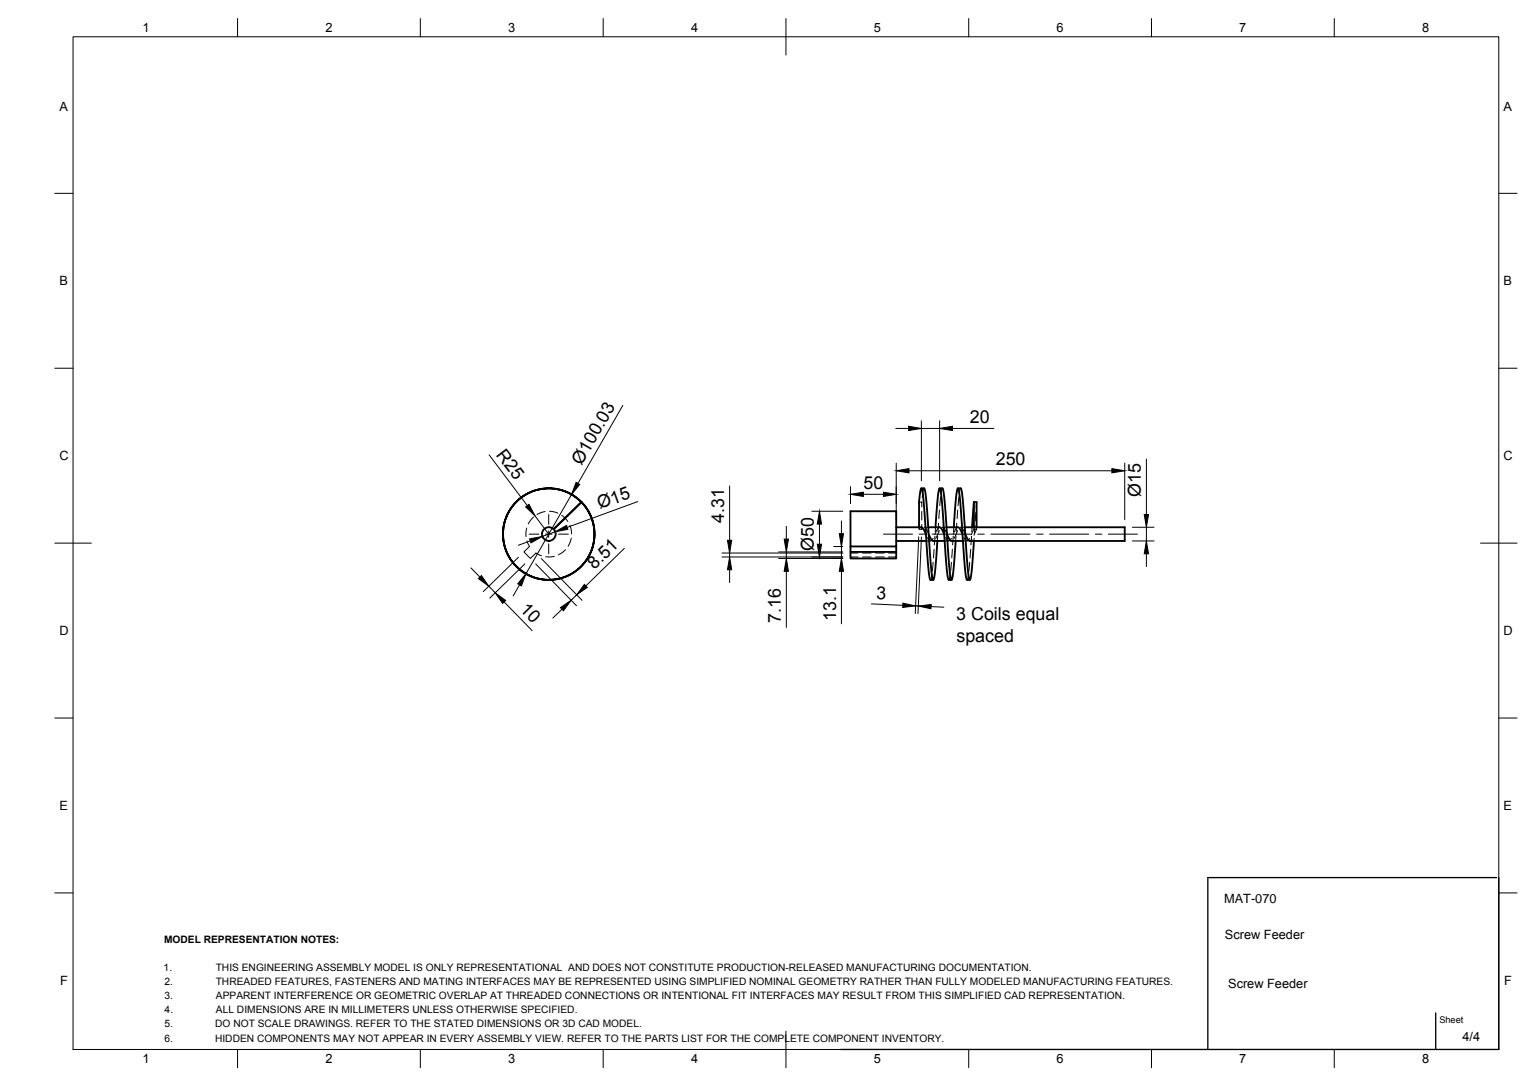
ISO-10303-21;
HEADER;
/* Generated by software containing ST-Developer
 * from STEP Tools, Inc. (www.steptools.com) 
 */

FILE_DESCRIPTION(
/* description */ (''),
/* implementation_level */ '2;1');

FILE_NAME(
/* name */ 'Screw Feeder.step',
/* time_stamp */ '2026-10-24T12:18:10-07:00',
/* author */ (''),
/* organization */ (''),
/* preprocessor_version */ 'ST-DEVELOPER v20.2',
/* originating_system */ 'Autodesk Translation Framework v15.15.0.0',
/* authorisation */ '');

FILE_SCHEMA (('AUTOMOTIVE_DESIGN { 1 0 10303 214 3 1 1 }'));
ENDSEC;

DATA;
#10=MECHANICAL_DESIGN_GEOMETRIC_PRESENTATION_REPRESENTATION('',(#39),#2858);
#19=(
BOUNDED_SURFACE()
B_SPLINE_SURFACE(1,2,((#1855,#1856,#1857,#1858,#1859,#1860,#1861,#1862,
#1863,#1864,#1865,#1866,#1867,#1868,#1869,#1870,#1871,#1872,#1873,#1874,
#1875,#1876,#1877,#1878,#1879,#1880,#1881,#1882,#1883,#1884,#1885,#1886,
#1887,#1888,#1889,#1890,#1891,#1892,#1893,#1894,#1895,#1896,#1897,#1898,
#1899,#1900,#1901,#1902,#1903,#1904,#1905,#1906,#1907,#1908,#1909,#1910,
#1911,#1912,#1913,#1914,#1915,#1916,#1917,#1918,#1919,#1920,#1921,#1922,
#1923,#1924,#1925,#1926,#1927,#1928,#1929,#1930,#1931,#1932,#1933,#1934,
#1935,#1936,#1937,#1938,#1939,#1940,#1941,#1942,#1943,#1944,#1945,#1946,
#1947,#1948,#1949,#1950,#1951,#1952,#1953,#1954,#1955,#1956,#1957,#1958,
#1959,#1960,#1961,#1962,#1963,#1964,#1965,#1966,#1967,#1968,#1969,#1970,
#1971,#1972,#1973,#1974,#1975),(#1976,#1977,#1978,#1979,#1980,#1981,#1982,
#1983,#1984,#1985,#1986,#1987,#1988,#1989,#1990,#1991,#1992,#1993,#1994,
#1995,#1996,#1997,#1998,#1999,#2000,#2001,#2002,#2003,#2004,#2005,#2006,
#2007,#2008,#2009,#2010,#2011,#2012,#2013,#2014,#2015,#2016,#2017,#2018,
#2019,#2020,#2021,#2022,#2023,#2024,#2025,#2026,#2027,#2028,#2029,#2030,
#2031,#2032,#2033,#2034,#2035,#2036,#2037,#2038,#2039,#2040,#2041,#2042,
#2043,#2044,#2045,#2046,#2047,#2048,#2049,#2050,#2051,#2052,#2053,#2054,
#2055,#2056,#2057,#2058,#2059,#2060,#2061,#2062,#2063,#2064,#2065,#2066,
#2067,#2068,#2069,#2070,#2071,#2072,#2073,#2074,#2075,#2076,#2077,#2078,
#2079,#2080,#2081,#2082,#2083,#2084,#2085,#2086,#2087,#2088,#2089,#2090,
#2091,#2092,#2093,#2094,#2095,#2096)),.UNSPECIFIED.,.F.,.F.,.F.)
B_SPLINE_SURFACE_WITH_KNOTS((2,2),(3,2,2,2,2,2,2,2,2,2,2,2,2,2,2,2,2,2,
2,2,2,2,2,2,2,2,2,2,2,2,2,2,2,2,2,2,2,2,2,2,2,2,2,2,2,2,2,2,2,2,2,2,2,2,
2,2,2,2,2,2,3),(0.,1.),(0.,0.0166666666666667,0.0333333333333333,0.05,0.0666666666666667,
0.0833333333333333,0.1,0.116666666666667,0.133333333333333,0.15,0.166666666666667,
0.183333333333333,0.2,0.216666666666667,0.233333333333333,0.25,0.266666666666667,
0.283333333333333,0.3,0.316666666666667,0.333333333333333,0.35,0.366666666666667,
0.383333333333333,0.4,0.416666666666667,0.433333333333333,0.45,0.466666666666667,
0.483333333333333,0.5,0.516666666666667,0.533333333333333,0.55,0.566666666666667,
0.583333333333333,0.6,0.616666666666667,0.633333333333333,0.65,0.666666666666667,
0.683333333333333,0.7,0.716666666666667,0.733333333333333,0.75,0.766666666666667,
0.783333333333333,0.8,0.816666666666667,0.833333333333333,0.85,0.866666666666667,
0.883333333333333,0.9,0.916666666666667,0.933333333333333,0.95,0.966666666666667,
0.983333333333333,1.),.UNSPECIFIED.)
GEOMETRIC_REPRESENTATION_ITEM()
RATIONAL_B_SPLINE_SURFACE(((1.,0.987688340595138,1.,0.987688340595138,1.,
0.987688340595138,1.,0.987688340595138,1.,0.987688340595138,1.,0.987688340595138,
1.,0.987688340595138,1.,0.987688340595138,1.,0.987688340595138,1.,0.987688340595138,
1.,0.987688340595138,1.,0.987688340595138,1.,0.987688340595138,1.,0.987688340595138,
1.,0.987688340595138,1.,0.987688340595138,1.,0.987688340595138,1.,0.987688340595138,
1.,0.987688340595138,1.,0.987688340595138,1.,0.987688340595138,1.,0.987688340595138,
1.,0.987688340595138,1.,0.987688340595138,1.,0.987688340595138,1.,0.987688340595138,
1.,0.987688340595138,1.,0.987688340595138,1.,0.987688340595138,1.,0.987688340595138,
1.,0.987688340595138,1.,0.987688340595138,1.,0.987688340595138,1.,0.987688340595138,
1.,0.987688340595138,1.,0.987688340595138,1.,0.987688340595138,1.,0.987688340595138,
1.,0.987688340595138,1.,0.987688340595138,1.,0.987688340595138,1.,0.987688340595138,
1.,0.987688340595138,1.,0.987688340595138,1.,0.987688340595138,1.,0.987688340595138,
1.,0.987688340595138,1.,0.987688340595138,1.,0.987688340595138,1.,0.987688340595138,
1.,0.987688340595138,1.,0.987688340595138,1.,0.987688340595138,1.,0.987688340595138,
1.,0.987688340595138,1.,0.987688340595138,1.,0.987688340595138,1.,0.987688340595138,
1.,0.987688340595138,1.,0.987688340595138,1.),(1.,0.987688340595138,1.,
0.987688340595138,1.,0.987688340595138,1.,0.987688340595138,1.,0.987688340595138,
1.,0.987688340595138,1.,0.987688340595138,1.,0.987688340595138,1.,0.987688340595138,
1.,0.987688340595138,1.,0.987688340595138,1.,0.987688340595138,1.,0.987688340595138,
1.,0.987688340595138,1.,0.987688340595138,1.,0.987688340595138,1.,0.987688340595138,
1.,0.987688340595138,1.,0.987688340595138,1.,0.987688340595138,1.,0.987688340595138,
1.,0.987688340595138,1.,0.987688340595138,1.,0.987688340595138,1.,0.987688340595138,
1.,0.987688340595138,1.,0.987688340595138,1.,0.987688340595138,1.,0.987688340595138,
1.,0.987688340595138,1.,0.987688340595138,1.,0.987688340595138,1.,0.987688340595138,
1.,0.987688340595138,1.,0.987688340595138,1.,0.987688340595138,1.,0.987688340595138,
1.,0.987688340595138,1.,0.987688340595138,1.,0.987688340595138,1.,0.987688340595138,
1.,0.987688340595138,1.,0.987688340595138,1.,0.987688340595138,1.,0.987688340595138,
1.,0.987688340595138,1.,0.987688340595138,1.,0.987688340595138,1.,0.987688340595138,
1.,0.987688340595138,1.,0.987688340595138,1.,0.987688340595138,1.,0.987688340595138,
1.,0.987688340595138,1.,0.987688340595138,1.,0.987688340595138,1.,0.987688340595138,
1.,0.987688340595138,1.,0.987688340595138,1.,0.987688340595138,1.)))
REPRESENTATION_ITEM('')
SURFACE()
);
#20=(
BOUNDED_SURFACE()
B_SPLINE_SURFACE(1,2,((#2218,#2219,#2220,#2221,#2222,#2223,#2224,#2225,
#2226,#2227,#2228,#2229,#2230,#2231,#2232,#2233,#2234,#2235,#2236,#2237,
#2238,#2239,#2240,#2241,#2242,#2243,#2244,#2245,#2246,#2247,#2248,#2249,
#2250,#2251,#2252,#2253,#2254,#2255,#2256,#2257,#2258,#2259,#2260,#2261,
#2262,#2263,#2264,#2265,#2266,#2267,#2268,#2269,#2270,#2271,#2272,#2273,
#2274,#2275,#2276,#2277,#2278,#2279,#2280,#2281,#2282,#2283,#2284,#2285,
#2286,#2287,#2288,#2289,#2290,#2291,#2292,#2293,#2294,#2295,#2296,#2297,
#2298,#2299,#2300,#2301,#2302,#2303,#2304,#2305,#2306,#2307,#2308,#2309,
#2310,#2311,#2312,#2313,#2314,#2315,#2316,#2317,#2318,#2319,#2320,#2321,
#2322,#2323,#2324,#2325,#2326,#2327,#2328,#2329,#2330,#2331,#2332,#2333,
#2334,#2335,#2336,#2337,#2338),(#2339,#2340,#2341,#2342,#2343,#2344,#2345,
#2346,#2347,#2348,#2349,#2350,#2351,#2352,#2353,#2354,#2355,#2356,#2357,
#2358,#2359,#2360,#2361,#2362,#2363,#2364,#2365,#2366,#2367,#2368,#2369,
#2370,#2371,#2372,#2373,#2374,#2375,#2376,#2377,#2378,#2379,#2380,#2381,
#2382,#2383,#2384,#2385,#2386,#2387,#2388,#2389,#2390,#2391,#2392,#2393,
#2394,#2395,#2396,#2397,#2398,#2399,#2400,#2401,#2402,#2403,#2404,#2405,
#2406,#2407,#2408,#2409,#2410,#2411,#2412,#2413,#2414,#2415,#2416,#2417,
#2418,#2419,#2420,#2421,#2422,#2423,#2424,#2425,#2426,#2427,#2428,#2429,
#2430,#2431,#2432,#2433,#2434,#2435,#2436,#2437,#2438,#2439,#2440,#2441,
#2442,#2443,#2444,#2445,#2446,#2447,#2448,#2449,#2450,#2451,#2452,#2453,
#2454,#2455,#2456,#2457,#2458,#2459)),.UNSPECIFIED.,.F.,.F.,.F.)
B_SPLINE_SURFACE_WITH_KNOTS((2,2),(3,2,2,2,2,2,2,2,2,2,2,2,2,2,2,2,2,2,
2,2,2,2,2,2,2,2,2,2,2,2,2,2,2,2,2,2,2,2,2,2,2,2,2,2,2,2,2,2,2,2,2,2,2,2,
2,2,2,2,2,2,3),(0.,1.),(0.,0.0166666666666667,0.0333333333333333,0.05,0.0666666666666667,
0.0833333333333333,0.1,0.116666666666667,0.133333333333333,0.15,0.166666666666667,
0.183333333333333,0.2,0.216666666666667,0.233333333333333,0.25,0.266666666666667,
0.283333333333333,0.3,0.316666666666667,0.333333333333333,0.35,0.366666666666667,
0.383333333333333,0.4,0.416666666666667,0.433333333333333,0.45,0.466666666666667,
0.483333333333333,0.5,0.516666666666667,0.533333333333333,0.55,0.566666666666667,
0.583333333333333,0.6,0.616666666666667,0.633333333333333,0.65,0.666666666666667,
0.683333333333333,0.7,0.716666666666667,0.733333333333333,0.75,0.766666666666667,
0.783333333333333,0.8,0.816666666666667,0.833333333333333,0.85,0.866666666666667,
0.883333333333333,0.9,0.916666666666667,0.933333333333333,0.95,0.966666666666667,
0.983333333333333,1.),.UNSPECIFIED.)
GEOMETRIC_REPRESENTATION_ITEM()
RATIONAL_B_SPLINE_SURFACE(((1.,0.987688340595138,1.,0.987688340595138,1.,
0.987688340595138,1.,0.987688340595138,1.,0.987688340595138,1.,0.987688340595138,
1.,0.987688340595138,1.,0.987688340595138,1.,0.987688340595138,1.,0.987688340595138,
1.,0.987688340595138,1.,0.987688340595138,1.,0.987688340595138,1.,0.987688340595138,
1.,0.987688340595138,1.,0.987688340595138,1.,0.987688340595138,1.,0.987688340595138,
1.,0.987688340595138,1.,0.987688340595138,1.,0.987688340595138,1.,0.987688340595138,
1.,0.987688340595138,1.,0.987688340595138,1.,0.987688340595138,1.,0.987688340595138,
1.,0.987688340595138,1.,0.987688340595138,1.,0.987688340595138,1.,0.987688340595138,
1.,0.987688340595138,1.,0.987688340595138,1.,0.987688340595138,1.,0.987688340595138,
1.,0.987688340595138,1.,0.987688340595138,1.,0.987688340595138,1.,0.987688340595138,
1.,0.987688340595138,1.,0.987688340595138,1.,0.987688340595138,1.,0.987688340595138,
1.,0.987688340595138,1.,0.987688340595138,1.,0.987688340595138,1.,0.987688340595138,
1.,0.987688340595138,1.,0.987688340595138,1.,0.987688340595138,1.,0.987688340595138,
1.,0.987688340595138,1.,0.987688340595138,1.,0.987688340595138,1.,0.987688340595138,
1.,0.987688340595138,1.,0.987688340595138,1.,0.987688340595138,1.,0.987688340595138,
1.,0.987688340595138,1.,0.987688340595138,1.),(1.,0.987688340595138,1.,
0.987688340595138,1.,0.987688340595138,1.,0.987688340595138,1.,0.987688340595138,
1.,0.987688340595138,1.,0.987688340595138,1.,0.987688340595138,1.,0.987688340595138,
1.,0.987688340595138,1.,0.987688340595138,1.,0.987688340595138,1.,0.987688340595138,
1.,0.987688340595138,1.,0.987688340595138,1.,0.987688340595138,1.,0.987688340595138,
1.,0.987688340595138,1.,0.987688340595138,1.,0.987688340595138,1.,0.987688340595138,
1.,0.987688340595138,1.,0.987688340595138,1.,0.987688340595138,1.,0.987688340595138,
1.,0.987688340595138,1.,0.987688340595138,1.,0.987688340595138,1.,0.987688340595138,
1.,0.987688340595138,1.,0.987688340595138,1.,0.987688340595138,1.,0.987688340595138,
1.,0.987688340595138,1.,0.987688340595138,1.,0.987688340595138,1.,0.987688340595138,
1.,0.987688340595138,1.,0.987688340595138,1.,0.987688340595138,1.,0.987688340595138,
1.,0.987688340595138,1.,0.987688340595138,1.,0.987688340595138,1.,0.987688340595138,
1.,0.987688340595138,1.,0.987688340595138,1.,0.987688340595138,1.,0.987688340595138,
1.,0.987688340595138,1.,0.987688340595138,1.,0.987688340595138,1.,0.987688340595138,
1.,0.987688340595138,1.,0.987688340595138,1.,0.987688340595138,1.,0.987688340595138,
1.,0.987688340595138,1.,0.987688340595138,1.,0.987688340595138,1.)))
REPRESENTATION_ITEM('')
SURFACE()
);
#21=(
BOUNDED_SURFACE()
B_SPLINE_SURFACE(1,2,((#2581,#2582,#2583,#2584,#2585,#2586,#2587,#2588,
#2589,#2590,#2591,#2592,#2593,#2594,#2595,#2596,#2597,#2598,#2599,#2600,
#2601,#2602,#2603,#2604,#2605,#2606,#2607,#2608,#2609,#2610,#2611,#2612,
#2613,#2614,#2615,#2616,#2617,#2618,#2619,#2620,#2621,#2622,#2623,#2624,
#2625,#2626,#2627,#2628,#2629,#2630,#2631,#2632,#2633,#2634,#2635,#2636,
#2637,#2638,#2639,#2640,#2641,#2642,#2643,#2644,#2645,#2646,#2647,#2648,
#2649,#2650,#2651,#2652,#2653,#2654,#2655,#2656,#2657,#2658,#2659,#2660,
#2661,#2662,#2663,#2664,#2665,#2666,#2667,#2668,#2669,#2670,#2671,#2672,
#2673,#2674,#2675,#2676,#2677,#2678,#2679,#2680,#2681,#2682,#2683,#2684,
#2685,#2686,#2687,#2688,#2689,#2690,#2691,#2692,#2693,#2694,#2695,#2696,
#2697,#2698,#2699,#2700,#2701),(#2702,#2703,#2704,#2705,#2706,#2707,#2708,
#2709,#2710,#2711,#2712,#2713,#2714,#2715,#2716,#2717,#2718,#2719,#2720,
#2721,#2722,#2723,#2724,#2725,#2726,#2727,#2728,#2729,#2730,#2731,#2732,
#2733,#2734,#2735,#2736,#2737,#2738,#2739,#2740,#2741,#2742,#2743,#2744,
#2745,#2746,#2747,#2748,#2749,#2750,#2751,#2752,#2753,#2754,#2755,#2756,
#2757,#2758,#2759,#2760,#2761,#2762,#2763,#2764,#2765,#2766,#2767,#2768,
#2769,#2770,#2771,#2772,#2773,#2774,#2775,#2776,#2777,#2778,#2779,#2780,
#2781,#2782,#2783,#2784,#2785,#2786,#2787,#2788,#2789,#2790,#2791,#2792,
#2793,#2794,#2795,#2796,#2797,#2798,#2799,#2800,#2801,#2802,#2803,#2804,
#2805,#2806,#2807,#2808,#2809,#2810,#2811,#2812,#2813,#2814,#2815,#2816,
#2817,#2818,#2819,#2820,#2821,#2822)),.UNSPECIFIED.,.F.,.F.,.F.)
B_SPLINE_SURFACE_WITH_KNOTS((2,2),(3,2,2,2,2,2,2,2,2,2,2,2,2,2,2,2,2,2,
2,2,2,2,2,2,2,2,2,2,2,2,2,2,2,2,2,2,2,2,2,2,2,2,2,2,2,2,2,2,2,2,2,2,2,2,
2,2,2,2,2,2,3),(0.,1.),(0.,0.0166666666666667,0.0333333333333333,0.05,0.0666666666666667,
0.0833333333333333,0.1,0.116666666666667,0.133333333333333,0.15,0.166666666666667,
0.183333333333333,0.2,0.216666666666667,0.233333333333333,0.25,0.266666666666667,
0.283333333333333,0.3,0.316666666666667,0.333333333333333,0.35,0.366666666666667,
0.383333333333333,0.4,0.416666666666667,0.433333333333333,0.45,0.466666666666667,
0.483333333333333,0.5,0.516666666666667,0.533333333333333,0.55,0.566666666666667,
0.583333333333333,0.6,0.616666666666667,0.633333333333333,0.65,0.666666666666667,
0.683333333333333,0.7,0.716666666666667,0.733333333333333,0.75,0.766666666666667,
0.783333333333333,0.8,0.816666666666667,0.833333333333333,0.85,0.866666666666667,
0.883333333333333,0.9,0.916666666666667,0.933333333333333,0.95,0.966666666666667,
0.983333333333333,1.),.UNSPECIFIED.)
GEOMETRIC_REPRESENTATION_ITEM()
RATIONAL_B_SPLINE_SURFACE(((1.,0.987688340595138,1.,0.987688340595138,1.,
0.987688340595138,1.,0.987688340595138,1.,0.987688340595138,1.,0.987688340595138,
1.,0.987688340595138,1.,0.987688340595138,1.,0.987688340595138,1.,0.987688340595138,
1.,0.987688340595138,1.,0.987688340595138,1.,0.987688340595138,1.,0.987688340595138,
1.,0.987688340595138,1.,0.987688340595138,1.,0.987688340595138,1.,0.987688340595138,
1.,0.987688340595138,1.,0.987688340595138,1.,0.987688340595138,1.,0.987688340595138,
1.,0.987688340595138,1.,0.987688340595138,1.,0.987688340595138,1.,0.987688340595138,
1.,0.987688340595138,1.,0.987688340595138,1.,0.987688340595138,1.,0.987688340595138,
1.,0.987688340595138,1.,0.987688340595138,1.,0.987688340595138,1.,0.987688340595138,
1.,0.987688340595138,1.,0.987688340595138,1.,0.987688340595138,1.,0.987688340595138,
1.,0.987688340595138,1.,0.987688340595138,1.,0.987688340595138,1.,0.987688340595138,
1.,0.987688340595138,1.,0.987688340595138,1.,0.987688340595138,1.,0.987688340595138,
1.,0.987688340595138,1.,0.987688340595138,1.,0.987688340595138,1.,0.987688340595138,
1.,0.987688340595138,1.,0.987688340595138,1.,0.987688340595138,1.,0.987688340595138,
1.,0.987688340595138,1.,0.987688340595138,1.,0.987688340595138,1.,0.987688340595138,
1.,0.987688340595138,1.,0.987688340595138,1.),(1.,0.987688340595138,1.,
0.987688340595138,1.,0.987688340595138,1.,0.987688340595138,1.,0.987688340595138,
1.,0.987688340595138,1.,0.987688340595138,1.,0.987688340595138,1.,0.987688340595138,
1.,0.987688340595138,1.,0.987688340595138,1.,0.987688340595138,1.,0.987688340595138,
1.,0.987688340595138,1.,0.987688340595138,1.,0.987688340595138,1.,0.987688340595138,
1.,0.987688340595138,1.,0.987688340595138,1.,0.987688340595138,1.,0.987688340595138,
1.,0.987688340595138,1.,0.987688340595138,1.,0.987688340595138,1.,0.987688340595138,
1.,0.987688340595138,1.,0.987688340595138,1.,0.987688340595138,1.,0.987688340595138,
1.,0.987688340595138,1.,0.987688340595138,1.,0.987688340595138,1.,0.987688340595138,
1.,0.987688340595138,1.,0.987688340595138,1.,0.987688340595138,1.,0.987688340595138,
1.,0.987688340595138,1.,0.987688340595138,1.,0.987688340595138,1.,0.987688340595138,
1.,0.987688340595138,1.,0.987688340595138,1.,0.987688340595138,1.,0.987688340595138,
1.,0.987688340595138,1.,0.987688340595138,1.,0.987688340595138,1.,0.987688340595138,
1.,0.987688340595138,1.,0.987688340595138,1.,0.987688340595138,1.,0.987688340595138,
1.,0.987688340595138,1.,0.987688340595138,1.,0.987688340595138,1.,0.987688340595138,
1.,0.987688340595138,1.,0.987688340595138,1.,0.987688340595138,1.)))
REPRESENTATION_ITEM('')
SURFACE()
);
#22=B_SPLINE_CURVE_WITH_KNOTS('',3,(#652,#653,#654,#655),.UNSPECIFIED.,
 .F.,.F.,(4,4),(-1.,-0.998645968698766),.UNSPECIFIED.);
#23=B_SPLINE_CURVE_WITH_KNOTS('',3,(#662,#663,#664,#665,#666,#667,#668,
#669,#670,#671,#672,#673,#674,#675,#676,#677,#678,#679,#680,#681,#682,#683,
#684,#685,#686,#687,#688,#689,#690,#691,#692,#693,#694,#695,#696,#697,#698,
#699,#700,#701,#702,#703,#704,#705,#706,#707,#708,#709,#710,#711,#712,#713,
#714,#715,#716,#717,#718,#719,#720,#721,#722,#723,#724,#725,#726,#727,#728,
#729,#730,#731,#732,#733,#734,#735,#736,#737,#738,#739,#740,#741,#742,#743,
#744,#745,#746,#747,#748,#749,#750,#751,#752,#753,#754,#755,#756,#757,#758,
#759,#760,#761,#762,#763,#764,#765,#766,#767,#768,#769,#770,#771,#772,#773,
#774,#775,#776,#777,#778,#779,#780,#781,#782,#783,#784,#785,#786,#787,#788,
#789,#790,#791,#792,#793,#794,#795,#796,#797,#798,#799,#800,#801,#802,#803,
#804,#805,#806,#807,#808,#809,#810,#811,#812,#813,#814,#815,#816,#817,#818,
#819,#820,#821,#822,#823,#824,#825,#826,#827,#828,#829,#830,#831,#832,#833,
#834,#835,#836,#837,#838,#839,#840,#841,#842,#843,#844,#845,#846,#847,#848,
#849,#850,#851,#852,#853,#854,#855,#856,#857,#858,#859,#860,#861,#862,#863,
#864,#865,#866,#867,#868,#869,#870,#871,#872,#873,#874,#875,#876,#877,#878,
#879,#880,#881,#882,#883,#884,#885,#886,#887,#888,#889,#890,#891,#892,#893,
#894,#895,#896,#897,#898,#899,#900,#901,#902,#903,#904,#905,#906,#907,#908,
#909,#910,#911,#912,#913,#914,#915,#916,#917,#918,#919,#920,#921,#922,#923,
#924,#925,#926,#927,#928,#929,#930,#931,#932,#933,#934,#935,#936,#937,#938,
#939,#940,#941,#942,#943,#944,#945,#946,#947,#948,#949,#950,#951,#952,#953,
#954,#955,#956,#957,#958,#959,#960,#961,#962,#963,#964,#965,#966,#967,#968,
#969,#970,#971,#972,#973,#974,#975,#976,#977,#978,#979,#980,#981,#982,#983,
#984,#985,#986,#987,#988,#989,#990,#991,#992,#993,#994,#995,#996,#997,#998,
#999,#1000,#1001,#1002,#1003,#1004,#1005,#1006,#1007,#1008,#1009,#1010,
#1011,#1012,#1013,#1014,#1015,#1016,#1017,#1018,#1019),.UNSPECIFIED.,.F.,
 .F.,(4,3,3,3,3,3,3,3,3,3,3,3,3,3,3,3,3,3,3,3,3,3,3,3,3,3,3,3,3,3,3,3,3,
3,3,3,3,3,3,3,3,3,3,3,3,3,3,3,3,3,3,3,3,3,3,3,3,3,3,3,3,3,3,3,3,3,3,3,3,
3,3,3,3,3,3,3,3,3,3,3,3,3,3,3,3,3,3,3,3,3,3,3,3,3,3,3,3,3,3,3,3,3,3,3,3,
3,3,3,3,3,3,3,3,3,3,3,3,3,3,4),(-0.331979302032099,-0.328745544947817,-0.325511126349503,
-0.322277581756429,-0.319042795051795,-0.316666666666667,-0.313432410645245,
-0.310074307983934,-0.306840488099785,-0.303607230746873,-0.300373105768056,
-0.3,-0.296765743978578,-0.293407641317267,-0.290173821433118,-0.286940564080179,
-0.283706439101408,-0.283333333333333,-0.280099077311897,-0.27674097465059,
-0.273507154766441,-0.270273897413541,-0.267039772434759,-0.266666666666667,
-0.263432410645244,-0.260074307983933,-0.25684048809978,-0.253607230746841,
-0.250373105768036,-0.25,-0.246765743978575,-0.243407641317264,-0.240173821433105,
-0.236940564080198,-0.233706439101398,-0.233333333333333,-0.230099077311924,
-0.22674097465061,-0.223507154766454,-0.220273897413536,-0.217039772434708,
-0.216666666666667,-0.213432410645268,-0.210074307983951,-0.206840488099798,
-0.203607230746877,-0.200373105768084,-0.2,-0.196765743978578,-0.193407641317267,
-0.190173821433123,-0.186940564080229,-0.183706439101414,-0.183333333333333,
-0.180099077311908,-0.176740974650597,-0.173507154766428,-0.170273897413483,
-0.167039772434678,-0.166666666666667,-0.163432410645259,-0.160074307983944,
-0.156840488099797,-0.153607230746853,-0.150373105768069,-0.15,-0.146765743978574,
-0.143407641317264,-0.140173821433101,-0.136940564080169,-0.133706439101386,
-0.133333333333333,-0.130099077311911,-0.1267409746506,-0.123507154766447,
-0.120273897413526,-0.117039772434722,-0.116666666666667,-0.113432410645241,
-0.110074307983931,-0.106840488099774,-0.103607230746858,-0.10037310576804,
-0.1,-0.0967657439785776,-0.0934076413172665,-0.0901738214331063,-0.0869405640801917,
-0.0837064391013879,-0.0833333333333334,-0.0800990773119075,-0.0767409746505973,
-0.0735071547664396,-0.0702738974135466,-0.0670397724347522,-0.0666666666666667,
-0.0634324106452447,-0.0600743079839336,-0.0568404880997839,-0.0536072307468639,
-0.0503731057680767,-0.05,-0.0467657439785748,-0.0434076413172644,-0.0401738214331216,
-0.0369405640801967,-0.033706439101418,-0.0333333333333333,-0.030099077311911,
-0.0267409746505999,-0.0235071547664523,-0.0202738974135343,-0.017039772434738,
-0.0166666666666667,-0.0134324106517174,-0.0100743318149406,-0.00684051195133032,
-0.00360725461687006,-0.000373129688631168,-9.53046099950368E-8),
 .UNSPECIFIED.);
#24=B_SPLINE_CURVE_WITH_KNOTS('',3,(#1066,#1067,#1068,#1069,#1070,#1071,
#1072,#1073,#1074,#1075,#1076,#1077,#1078,#1079,#1080,#1081,#1082,#1083,
#1084,#1085,#1086,#1087,#1088,#1089,#1090,#1091,#1092,#1093,#1094,#1095,
#1096,#1097,#1098,#1099,#1100,#1101,#1102,#1103,#1104,#1105,#1106,#1107,
#1108,#1109,#1110,#1111,#1112,#1113,#1114,#1115,#1116,#1117,#1118,#1119,
#1120,#1121,#1122,#1123,#1124,#1125,#1126,#1127,#1128,#1129,#1130,#1131,
#1132,#1133,#1134,#1135,#1136,#1137,#1138,#1139,#1140,#1141,#1142,#1143,
#1144,#1145,#1146,#1147,#1148,#1149,#1150,#1151,#1152,#1153,#1154,#1155,
#1156,#1157,#1158,#1159,#1160,#1161,#1162,#1163,#1164,#1165,#1166,#1167,
#1168,#1169,#1170,#1171,#1172,#1173,#1174,#1175,#1176,#1177,#1178,#1179,
#1180,#1181,#1182,#1183,#1184,#1185,#1186,#1187,#1188,#1189,#1190,#1191,
#1192,#1193,#1194,#1195,#1196,#1197,#1198,#1199,#1200,#1201,#1202,#1203,
#1204,#1205,#1206,#1207,#1208,#1209,#1210,#1211,#1212,#1213,#1214,#1215,
#1216,#1217,#1218,#1219,#1220,#1221,#1222,#1223,#1224,#1225,#1226,#1227,
#1228,#1229,#1230,#1231,#1232,#1233,#1234,#1235,#1236,#1237,#1238,#1239,
#1240,#1241,#1242,#1243,#1244,#1245,#1246,#1247,#1248,#1249,#1250,#1251,
#1252,#1253,#1254,#1255,#1256,#1257,#1258,#1259,#1260,#1261,#1262,#1263,
#1264,#1265,#1266,#1267,#1268,#1269,#1270,#1271,#1272,#1273,#1274,#1275,
#1276,#1277,#1278,#1279,#1280,#1281,#1282,#1283,#1284,#1285,#1286,#1287,
#1288,#1289,#1290,#1291,#1292,#1293,#1294,#1295,#1296,#1297,#1298,#1299,
#1300,#1301,#1302,#1303,#1304,#1305,#1306,#1307,#1308,#1309,#1310,#1311,
#1312,#1313,#1314,#1315,#1316,#1317,#1318,#1319,#1320,#1321,#1322,#1323,
#1324,#1325,#1326,#1327,#1328,#1329,#1330,#1331,#1332,#1333,#1334,#1335,
#1336,#1337,#1338,#1339,#1340,#1341,#1342,#1343,#1344,#1345,#1346,#1347,
#1348,#1349,#1350,#1351,#1352,#1353,#1354,#1355,#1356,#1357,#1358,#1359,
#1360,#1361,#1362,#1363,#1364,#1365,#1366,#1367,#1368,#1369,#1370,#1371,
#1372,#1373,#1374,#1375,#1376,#1377,#1378,#1379,#1380,#1381,#1382,#1383,
#1384,#1385,#1386,#1387,#1388,#1389,#1390,#1391,#1392,#1393,#1394,#1395,
#1396,#1397,#1398,#1399,#1400,#1401,#1402,#1403,#1404,#1405,#1406,#1407,
#1408,#1409,#1410,#1411,#1412,#1413,#1414,#1415,#1416,#1417,#1418,#1419,
#1420,#1421,#1422,#1423,#1424,#1425,#1426),.UNSPECIFIED.,.F.,.F.,(4,3,3,
3,3,3,3,3,3,3,3,3,3,3,3,3,3,3,3,3,3,3,3,3,3,3,3,3,3,3,3,3,3,3,3,3,3,3,3,
3,3,3,3,3,3,3,3,3,3,3,3,3,3,3,3,3,3,3,3,3,3,3,3,3,3,3,3,3,3,3,3,3,3,3,3,
3,3,3,3,3,3,3,3,3,3,3,3,3,3,3,3,3,3,3,3,3,3,3,3,3,3,3,3,3,3,3,3,3,3,3,3,
3,3,3,3,3,3,3,3,3,4),(-0.665312635365433,-0.662078878281142,-0.658844459682826,
-0.655610915089758,-0.652376128385123,-0.65,-0.646765743978579,-0.643407641317267,
-0.640173821433118,-0.636940564080195,-0.633706439101402,-0.633333333333333,
-0.630099077311912,-0.626740974650601,-0.623507154766448,-0.620273897413523,
-0.617039772434729,-0.616666666666667,-0.613432410645243,-0.610074307983932,
-0.60684048809978,-0.603607230746855,-0.60037310576806,-0.6,-0.596765743978578,
-0.593407641317267,-0.590173821433114,-0.586940564080189,-0.583706439101395,
-0.583333333333333,-0.580099077311911,-0.5767409746506,-0.573507154766447,
-0.570273897413521,-0.567039772434727,-0.566666666666667,-0.563432410645245,
-0.560074307983934,-0.556840488099781,-0.553607230746856,-0.550373105768065,
-0.55,-0.546765743978579,-0.543407641317267,-0.540173821433115,-0.536940564080189,
-0.533706439101384,-0.533333333333333,-0.530099077311911,-0.5267409746506,
-0.523507154766446,-0.52027389741352,-0.517039772434727,-0.516666666666667,
-0.513432410645245,-0.510074307983934,-0.506840488099781,-0.503607230746855,
-0.500373105768063,-0.5,-0.496765743978578,-0.493407641317267,-0.490173821433103,
-0.486940564080178,-0.483706439101384,-0.483333333333333,-0.480099077311911,
-0.4767409746506,-0.473507154766447,-0.47027389741351,-0.467039772434717,
-0.466666666666667,-0.463432410645245,-0.460074307983933,-0.456840488099777,
-0.453607230746852,-0.450373105768059,-0.45,-0.446765743978577,-0.443407641317266,
-0.440173821433109,-0.43694056408017,-0.433706439101377,-0.433333333333333,
-0.430099077311911,-0.4267409746506,-0.423507154766447,-0.420273897413509,
-0.417039772434716,-0.416666666666667,-0.413432410645244,-0.410074307983933,
-0.40684048809978,-0.403607230746867,-0.400373105768075,-0.4,-0.396765743978578,
-0.393407641317267,-0.390173821433118,-0.386940564080206,-0.383706439101414,
-0.383333333333333,-0.380099077311912,-0.376740974650601,-0.373507154766456,
-0.370273897413568,-0.367039772434754,-0.366666666666667,-0.363432410645244,
-0.360074307983933,-0.356840488099784,-0.353607230746845,-0.350373105768042,
-0.35,-0.346765743978578,-0.343407641317267,-0.34017382143311,-0.336940564080171,
-0.333706439101378,-0.333333333333333,-0.331979302032099),.UNSPECIFIED.);
#25=B_SPLINE_CURVE_WITH_KNOTS('',3,(#1472,#1473,#1474,#1475,#1476,#1477,
#1478,#1479,#1480,#1481,#1482,#1483,#1484,#1485,#1486,#1487,#1488,#1489,
#1490,#1491,#1492,#1493,#1494,#1495,#1496,#1497,#1498,#1499,#1500,#1501,
#1502,#1503,#1504,#1505,#1506,#1507,#1508,#1509,#1510,#1511,#1512,#1513,
#1514,#1515,#1516,#1517,#1518,#1519,#1520,#1521,#1522,#1523,#1524,#1525,
#1526,#1527,#1528,#1529,#1530,#1531,#1532,#1533,#1534,#1535,#1536,#1537,
#1538,#1539,#1540,#1541,#1542,#1543,#1544,#1545,#1546,#1547,#1548,#1549,
#1550,#1551,#1552,#1553,#1554,#1555,#1556,#1557,#1558,#1559,#1560,#1561,
#1562,#1563,#1564,#1565,#1566,#1567,#1568,#1569,#1570,#1571,#1572,#1573,
#1574,#1575,#1576,#1577,#1578,#1579,#1580,#1581,#1582,#1583,#1584,#1585,
#1586,#1587,#1588,#1589,#1590,#1591,#1592,#1593,#1594,#1595,#1596,#1597,
#1598,#1599,#1600,#1601,#1602,#1603,#1604,#1605,#1606,#1607,#1608,#1609,
#1610,#1611,#1612,#1613,#1614,#1615,#1616,#1617,#1618,#1619,#1620,#1621,
#1622,#1623,#1624,#1625,#1626,#1627,#1628,#1629,#1630,#1631,#1632,#1633,
#1634,#1635,#1636,#1637,#1638,#1639,#1640,#1641,#1642,#1643,#1644,#1645,
#1646,#1647,#1648,#1649,#1650,#1651,#1652,#1653,#1654,#1655,#1656,#1657,
#1658,#1659,#1660,#1661,#1662,#1663,#1664,#1665,#1666,#1667,#1668,#1669,
#1670,#1671,#1672,#1673,#1674,#1675,#1676,#1677,#1678,#1679,#1680,#1681,
#1682,#1683,#1684,#1685,#1686,#1687,#1688,#1689,#1690,#1691,#1692,#1693,
#1694,#1695,#1696,#1697,#1698,#1699,#1700,#1701,#1702,#1703,#1704,#1705,
#1706,#1707,#1708,#1709,#1710,#1711,#1712,#1713,#1714,#1715,#1716,#1717,
#1718,#1719,#1720,#1721,#1722,#1723,#1724,#1725,#1726,#1727,#1728,#1729,
#1730,#1731,#1732,#1733,#1734,#1735,#1736,#1737,#1738,#1739,#1740,#1741,
#1742,#1743,#1744,#1745,#1746,#1747,#1748,#1749,#1750,#1751,#1752,#1753,
#1754,#1755,#1756,#1757,#1758,#1759,#1760,#1761,#1762,#1763,#1764,#1765,
#1766,#1767,#1768,#1769,#1770,#1771,#1772,#1773,#1774,#1775,#1776,#1777,
#1778,#1779,#1780,#1781,#1782,#1783,#1784,#1785,#1786,#1787,#1788,#1789,
#1790,#1791,#1792,#1793,#1794,#1795,#1796,#1797,#1798,#1799,#1800,#1801,
#1802,#1803,#1804,#1805,#1806,#1807,#1808,#1809,#1810,#1811,#1812,#1813,
#1814,#1815,#1816,#1817,#1818,#1819,#1820,#1821,#1822,#1823,#1824,#1825,
#1826,#1827,#1828,#1829,#1830,#1831,#1832),.UNSPECIFIED.,.F.,.F.,(4,3,3,
3,3,3,3,3,3,3,3,3,3,3,3,3,3,3,3,3,3,3,3,3,3,3,3,3,3,3,3,3,3,3,3,3,3,3,3,
3,3,3,3,3,3,3,3,3,3,3,3,3,3,3,3,3,3,3,3,3,3,3,3,3,3,3,3,3,3,3,3,3,3,3,3,
3,3,3,3,3,3,3,3,3,3,3,3,3,3,3,3,3,3,3,3,3,3,3,3,3,3,3,3,3,3,3,3,3,3,3,3,
3,3,3,3,3,3,3,3,3,4),(-0.998645968698766,-0.995412211614476,-0.99217779301616,
-0.988944248423087,-0.985709461718452,-0.983333333333333,-0.980099077311911,
-0.9767409746506,-0.973507154766447,-0.970273897413519,-0.967039772434726,
-0.966666666666667,-0.963432410645243,-0.960074307983932,-0.956840488099779,
-0.953607230746854,-0.950373105768062,-0.95,-0.946765743978577,-0.943407641317266,
-0.940173821433113,-0.936940564080185,-0.933706439101392,-0.933333333333333,
-0.930099077311911,-0.9267409746506,-0.923507154766446,-0.92027389741352,
-0.917039772434728,-0.916666666666667,-0.913432410645244,-0.910074307983933,
-0.90684048809978,-0.903607230746854,-0.90037310576806,-0.9,-0.896765743978578,
-0.893407641317267,-0.890173821433115,-0.886940564080189,-0.883706439101396,
-0.883333333333333,-0.880099077311911,-0.8767409746506,-0.873507154766449,
-0.870273897413525,-0.867039772434733,-0.866666666666667,-0.863432410645245,
-0.860074307983934,-0.856840488099781,-0.853607230746854,-0.850373105768058,
-0.85,-0.846765743978578,-0.843407641317267,-0.840173821433114,-0.836940564080188,
-0.833706439101395,-0.833333333333333,-0.830099077311911,-0.8267409746506,
-0.823507154766447,-0.820273897413526,-0.817039772434731,-0.816666666666667,
-0.81343241064524,-0.81007430798393,-0.806840488099777,-0.803607230746853,
-0.800373105768059,-0.8,-0.796765743978579,-0.793407641317267,-0.790173821433115,
-0.786940564080183,-0.783706439101388,-0.783333333333333,-0.780099077311911,
-0.7767409746506,-0.773507154766446,-0.770273897413509,-0.767039772434712,
-0.766666666666667,-0.763432410645249,-0.760074307983936,-0.756840488099782,
-0.753607230746868,-0.75037310576807,-0.75,-0.746765743978578,-0.743407641317267,
-0.740173821433118,-0.736940564080168,-0.733706439101356,-0.733333333333333,
-0.730099077311911,-0.7267409746506,-0.723507154766451,-0.720273897413524,
-0.717039772434739,-0.716666666666667,-0.713432410645237,-0.710074307983928,
-0.706840488099775,-0.703607230746849,-0.700373105768067,-0.7,-0.69676574397857,
-0.693407641317261,-0.690173821433107,-0.686940564080183,-0.683706439101389,
-0.683333333333333,-0.680099077311912,-0.6767409746506,-0.673507154766448,
-0.670273897413522,-0.667039772434727,-0.666666666666667,-0.665312635365433),
 .UNSPECIFIED.);
#26=B_SPLINE_CURVE_WITH_KNOTS('',3,(#1835,#1836,#1837,#1838,#1839,#1840),
 .UNSPECIFIED.,.F.,.F.,(4,2,4),(-4.25163970020424,-2.12588055073164,0.),
 .UNSPECIFIED.);
#27=B_SPLINE_CURVE_WITH_KNOTS('',3,(#1846,#1847,#1848,#1849,#1850,#1851),
 .UNSPECIFIED.,.F.,.F.,(4,2,4),(-4.25163970020424,-2.1257591494726,0.),
 .UNSPECIFIED.);
#28=(
BOUNDED_CURVE()
B_SPLINE_CURVE(2,(#600,#601,#602,#603,#604,#605,#606,#607,#608,#609,#610,
#611,#612,#613,#614,#615,#616,#617,#618,#619,#620,#621,#622,#623,#624,#625,
#626,#627,#628,#629,#630,#631,#632,#633,#634,#635,#636,#637,#638,#639,#640,
#641,#642),.UNSPECIFIED.,.F.,.F.)
B_SPLINE_CURVE_WITH_KNOTS((3,2,2,2,2,2,2,2,2,2,2,2,2,2,2,2,2,2,2,2,2,3),
(1.82334519084262E-6,0.0166666666666667,0.0333333333333333,0.05,0.0666666666666667,
0.0833333333333333,0.1,0.116666666666667,0.133333333333333,0.15,0.166666666666667,
0.183333333333333,0.2,0.216666666666667,0.233333333333333,0.25,0.266666666666667,
0.283333333333333,0.3,0.316666666666667,0.333333333333333,0.333335156678524),
 .UNSPECIFIED.)
CURVE()
GEOMETRIC_REPRESENTATION_ITEM()
RATIONAL_B_SPLINE_CURVE((0.999997306486108,0.987689687499436,1.,0.987688340595138,
1.,0.987688340595138,1.,0.987688340595138,1.,0.987688340595138,1.,0.987688340595138,
1.,0.987688340595138,1.,0.987688340595138,1.,0.987688340595138,1.,0.987688340595138,
1.,0.987688340595138,1.,0.987688340595138,1.,0.987688340595138,1.,0.987688340595138,
1.,0.987688340595138,1.,0.987688340595138,1.,0.987688340595138,1.,0.987688340595138,
1.,0.987688340595138,1.,0.987688340595138,1.,0.999998653095702,0.999997306486109))
REPRESENTATION_ITEM('')
);
#29=(
BOUNDED_CURVE()
B_SPLINE_CURVE(2,(#647,#648,#649),.UNSPECIFIED.,.F.,.F.)
B_SPLINE_CURVE_WITH_KNOTS((3,3),(0.,1.82334519084262E-6),.UNSPECIFIED.)
CURVE()
GEOMETRIC_REPRESENTATION_ITEM()
RATIONAL_B_SPLINE_CURVE((1.,0.999998653095702,0.999997306486108))
REPRESENTATION_ITEM('')
);
#30=(
BOUNDED_CURVE()
B_SPLINE_CURVE(2,(#1023,#1024,#1025,#1026,#1027,#1028,#1029,#1030,#1031,
#1032,#1033,#1034,#1035,#1036,#1037,#1038,#1039,#1040,#1041,#1042,#1043,
#1044,#1045,#1046,#1047,#1048,#1049,#1050,#1051,#1052,#1053,#1054,#1055,
#1056,#1057,#1058,#1059,#1060,#1061,#1062,#1063),.UNSPECIFIED.,.F.,.F.)
B_SPLINE_CURVE_WITH_KNOTS((3,2,2,2,2,2,2,2,2,2,2,2,2,2,2,2,2,2,2,2,3),(0.666668490011857,
0.683333333333333,0.7,0.716666666666667,0.733333333333333,0.75,0.766666666666667,
0.783333333333333,0.8,0.816666666666667,0.833333333333333,0.85,0.866666666666667,
0.883333333333333,0.9,0.916666666666667,0.933333333333333,0.95,0.966666666666667,
0.983333333333333,1.),.UNSPECIFIED.)
CURVE()
GEOMETRIC_REPRESENTATION_ITEM()
RATIONAL_B_SPLINE_CURVE((0.999997306486109,0.987689687499436,1.,0.987688340595138,
1.,0.987688340595138,1.,0.987688340595138,1.,0.987688340595138,1.,0.987688340595138,
1.,0.987688340595138,1.,0.987688340595138,1.,0.987688340595138,1.,0.987688340595138,
1.,0.987688340595138,1.,0.987688340595138,1.,0.987688340595138,1.,0.987688340595138,
1.,0.987688340595138,1.,0.987688340595138,1.,0.987688340595138,1.,0.987688340595138,
1.,0.987688340595138,1.,0.987688340595138,1.))
REPRESENTATION_ITEM('')
);
#31=(
BOUNDED_CURVE()
B_SPLINE_CURVE(2,(#1429,#1430,#1431,#1432,#1433,#1434,#1435,#1436,#1437,
#1438,#1439,#1440,#1441,#1442,#1443,#1444,#1445,#1446,#1447,#1448,#1449,
#1450,#1451,#1452,#1453,#1454,#1455,#1456,#1457,#1458,#1459,#1460,#1461,
#1462,#1463,#1464,#1465,#1466,#1467,#1468,#1469,#1470,#1471),
 .UNSPECIFIED.,.F.,.F.)
B_SPLINE_CURVE_WITH_KNOTS((3,2,2,2,2,2,2,2,2,2,2,2,2,2,2,2,2,2,2,2,2,3),
(0.333335156678524,0.35,0.366666666666667,0.383333333333333,0.4,0.416666666666667,
0.433333333333333,0.45,0.466666666666667,0.483333333333333,0.5,0.516666666666667,
0.533333333333333,0.55,0.566666666666667,0.583333333333333,0.6,0.616666666666667,
0.633333333333333,0.65,0.666666666666667,0.666668490011857),
 .UNSPECIFIED.)
CURVE()
GEOMETRIC_REPRESENTATION_ITEM()
RATIONAL_B_SPLINE_CURVE((0.999997306486109,0.987689687499436,1.,0.987688340595138,
1.,0.987688340595138,1.,0.987688340595138,1.,0.987688340595138,1.,0.987688340595138,
1.,0.987688340595138,1.,0.987688340595138,1.,0.987688340595138,1.,0.987688340595138,
1.,0.987688340595138,1.,0.987688340595138,1.,0.987688340595138,1.,0.987688340595138,
1.,0.987688340595138,1.,0.987688340595138,1.,0.987688340595138,1.,0.987688340595138,
1.,0.987688340595138,1.,0.987688340595138,1.,0.999998653095702,0.999997306486109))
REPRESENTATION_ITEM('')
);
#32=(
BOUNDED_CURVE()
B_SPLINE_CURVE(2,(#2097,#2098,#2099,#2100,#2101,#2102,#2103,#2104,#2105,
#2106,#2107,#2108,#2109,#2110,#2111,#2112,#2113,#2114,#2115,#2116,#2117,
#2118,#2119,#2120,#2121,#2122,#2123,#2124,#2125,#2126,#2127,#2128,#2129,
#2130,#2131,#2132,#2133,#2134,#2135,#2136,#2137,#2138,#2139,#2140,#2141,
#2142,#2143,#2144,#2145,#2146,#2147,#2148,#2149,#2150,#2151,#2152,#2153,
#2154,#2155,#2156,#2157,#2158,#2159,#2160,#2161,#2162,#2163,#2164,#2165,
#2166,#2167,#2168,#2169,#2170,#2171,#2172,#2173,#2174,#2175,#2176,#2177,
#2178,#2179,#2180,#2181,#2182,#2183,#2184,#2185,#2186,#2187,#2188,#2189,
#2190,#2191,#2192,#2193,#2194,#2195,#2196,#2197,#2198,#2199,#2200,#2201,
#2202,#2203,#2204,#2205,#2206,#2207,#2208,#2209,#2210,#2211,#2212,#2213,
#2214,#2215,#2216,#2217),.UNSPECIFIED.,.F.,.F.)
B_SPLINE_CURVE_WITH_KNOTS((3,2,2,2,2,2,2,2,2,2,2,2,2,2,2,2,2,2,2,2,2,2,
2,2,2,2,2,2,2,2,2,2,2,2,2,2,2,2,2,2,2,2,2,2,2,2,2,2,2,2,2,2,2,2,2,2,2,2,
2,2,3),(0.,0.0166666666666667,0.0333333333333333,0.05,0.0666666666666667,
0.0833333333333333,0.1,0.116666666666667,0.133333333333333,0.15,0.166666666666667,
0.183333333333333,0.2,0.216666666666667,0.233333333333333,0.25,0.266666666666667,
0.283333333333333,0.3,0.316666666666667,0.333333333333333,0.35,0.366666666666667,
0.383333333333333,0.4,0.416666666666667,0.433333333333333,0.45,0.466666666666667,
0.483333333333333,0.5,0.516666666666667,0.533333333333333,0.55,0.566666666666667,
0.583333333333333,0.6,0.616666666666667,0.633333333333333,0.65,0.666666666666667,
0.683333333333333,0.7,0.716666666666667,0.733333333333333,0.75,0.766666666666667,
0.783333333333333,0.8,0.816666666666667,0.833333333333333,0.85,0.866666666666667,
0.883333333333333,0.9,0.916666666666667,0.933333333333333,0.95,0.966666666666667,
0.983333333333333,1.),.UNSPECIFIED.)
CURVE()
GEOMETRIC_REPRESENTATION_ITEM()
RATIONAL_B_SPLINE_CURVE((1.,0.987688340595138,1.,0.987688340595138,1.,0.987688340595138,
1.,0.987688340595138,1.,0.987688340595138,1.,0.987688340595138,1.,0.987688340595138,
1.,0.987688340595138,1.,0.987688340595138,1.,0.987688340595138,1.,0.987688340595138,
1.,0.987688340595138,1.,0.987688340595138,1.,0.987688340595138,1.,0.987688340595138,
1.,0.987688340595138,1.,0.987688340595138,1.,0.987688340595138,1.,0.987688340595138,
1.,0.987688340595138,1.,0.987688340595138,1.,0.987688340595138,1.,0.987688340595138,
1.,0.987688340595138,1.,0.987688340595138,1.,0.987688340595138,1.,0.987688340595138,
1.,0.987688340595138,1.,0.987688340595138,1.,0.987688340595138,1.,0.987688340595138,
1.,0.987688340595138,1.,0.987688340595138,1.,0.987688340595138,1.,0.987688340595138,
1.,0.987688340595138,1.,0.987688340595138,1.,0.987688340595138,1.,0.987688340595138,
1.,0.987688340595138,1.,0.987688340595138,1.,0.987688340595138,1.,0.987688340595138,
1.,0.987688340595138,1.,0.987688340595138,1.,0.987688340595138,1.,0.987688340595138,
1.,0.987688340595138,1.,0.987688340595138,1.,0.987688340595138,1.,0.987688340595138,
1.,0.987688340595138,1.,0.987688340595138,1.,0.987688340595138,1.,0.987688340595138,
1.,0.987688340595138,1.,0.987688340595138,1.,0.987688340595138,1.,0.987688340595138,
1.,0.987688340595138,1.))
REPRESENTATION_ITEM('')
);
#33=(
BOUNDED_CURVE()
B_SPLINE_CURVE(2,(#2460,#2461,#2462,#2463,#2464,#2465,#2466,#2467,#2468,
#2469,#2470,#2471,#2472,#2473,#2474,#2475,#2476,#2477,#2478,#2479,#2480,
#2481,#2482,#2483,#2484,#2485,#2486,#2487,#2488,#2489,#2490,#2491,#2492,
#2493,#2494,#2495,#2496,#2497,#2498,#2499,#2500,#2501,#2502,#2503,#2504,
#2505,#2506,#2507,#2508,#2509,#2510,#2511,#2512,#2513,#2514,#2515,#2516,
#2517,#2518,#2519,#2520,#2521,#2522,#2523,#2524,#2525,#2526,#2527,#2528,
#2529,#2530,#2531,#2532,#2533,#2534,#2535,#2536,#2537,#2538,#2539,#2540,
#2541,#2542,#2543,#2544,#2545,#2546,#2547,#2548,#2549,#2550,#2551,#2552,
#2553,#2554,#2555,#2556,#2557,#2558,#2559,#2560,#2561,#2562,#2563,#2564,
#2565,#2566,#2567,#2568,#2569,#2570,#2571,#2572,#2573,#2574,#2575,#2576,
#2577,#2578,#2579,#2580),.UNSPECIFIED.,.F.,.F.)
B_SPLINE_CURVE_WITH_KNOTS((3,2,2,2,2,2,2,2,2,2,2,2,2,2,2,2,2,2,2,2,2,2,
2,2,2,2,2,2,2,2,2,2,2,2,2,2,2,2,2,2,2,2,2,2,2,2,2,2,2,2,2,2,2,2,2,2,2,2,
2,2,3),(0.,0.0166666666666667,0.0333333333333333,0.05,0.0666666666666667,
0.0833333333333333,0.1,0.116666666666667,0.133333333333333,0.15,0.166666666666667,
0.183333333333333,0.2,0.216666666666667,0.233333333333333,0.25,0.266666666666667,
0.283333333333333,0.3,0.316666666666667,0.333333333333333,0.35,0.366666666666667,
0.383333333333333,0.4,0.416666666666667,0.433333333333333,0.45,0.466666666666667,
0.483333333333333,0.5,0.516666666666667,0.533333333333333,0.55,0.566666666666667,
0.583333333333333,0.6,0.616666666666667,0.633333333333333,0.65,0.666666666666667,
0.683333333333333,0.7,0.716666666666667,0.733333333333333,0.75,0.766666666666667,
0.783333333333333,0.8,0.816666666666667,0.833333333333333,0.85,0.866666666666667,
0.883333333333333,0.9,0.916666666666667,0.933333333333333,0.95,0.966666666666667,
0.983333333333333,1.),.UNSPECIFIED.)
CURVE()
GEOMETRIC_REPRESENTATION_ITEM()
RATIONAL_B_SPLINE_CURVE((1.,0.987688340595138,1.,0.987688340595138,1.,0.987688340595138,
1.,0.987688340595138,1.,0.987688340595138,1.,0.987688340595138,1.,0.987688340595138,
1.,0.987688340595138,1.,0.987688340595138,1.,0.987688340595138,1.,0.987688340595138,
1.,0.987688340595138,1.,0.987688340595138,1.,0.987688340595138,1.,0.987688340595138,
1.,0.987688340595138,1.,0.987688340595138,1.,0.987688340595138,1.,0.987688340595138,
1.,0.987688340595138,1.,0.987688340595138,1.,0.987688340595138,1.,0.987688340595138,
1.,0.987688340595138,1.,0.987688340595138,1.,0.987688340595138,1.,0.987688340595138,
1.,0.987688340595138,1.,0.987688340595138,1.,0.987688340595138,1.,0.987688340595138,
1.,0.987688340595138,1.,0.987688340595138,1.,0.987688340595138,1.,0.987688340595138,
1.,0.987688340595138,1.,0.987688340595138,1.,0.987688340595138,1.,0.987688340595138,
1.,0.987688340595138,1.,0.987688340595138,1.,0.987688340595138,1.,0.987688340595138,
1.,0.987688340595138,1.,0.987688340595138,1.,0.987688340595138,1.,0.987688340595138,
1.,0.987688340595138,1.,0.987688340595138,1.,0.987688340595138,1.,0.987688340595138,
1.,0.987688340595138,1.,0.987688340595138,1.,0.987688340595138,1.,0.987688340595138,
1.,0.987688340595138,1.,0.987688340595138,1.,0.987688340595138,1.,0.987688340595138,
1.,0.987688340595138,1.))
REPRESENTATION_ITEM('')
);
#35=SHAPE_REPRESENTATION_RELATIONSHIP('SRR','None',#2873,#37);
#37=ADVANCED_BREP_SHAPE_REPRESENTATION('',(#41),#2857);
#39=STYLED_ITEM('',(#2890),#41);
#41=MANIFOLD_SOLID_BREP('Screw Feeder',#390);
#45=CYLINDRICAL_SURFACE('',#435,7.5);
#46=CYLINDRICAL_SURFACE('',#438,7.5);
#47=CYLINDRICAL_SURFACE('',#442,7.5);
#48=CYLINDRICAL_SURFACE('',#445,25.);
#54=LINE('',#598,#77);
#55=LINE('',#644,#78);
#56=LINE('',#660,#79);
#57=LINE('',#1065,#80);
#58=LINE('',#1842,#81);
#59=LINE('',#1843,#82);
#60=LINE('',#1853,#83);
#61=LINE('',#1854,#84);
#62=LINE('',#2828,#85);
#63=LINE('',#2831,#86);
#64=LINE('',#2834,#87);
#65=LINE('',#2836,#88);
#66=LINE('',#2837,#89);
#67=LINE('',#2840,#90);
#68=LINE('',#2842,#91);
#69=LINE('',#2843,#92);
#70=LINE('',#2845,#93);
#71=LINE('',#2846,#94);
#77=VECTOR('',#504,7.5);
#78=VECTOR('',#505,7.5);
#79=VECTOR('',#514,7.5);
#80=VECTOR('',#517,7.5);
#81=VECTOR('',#524,42.5163970020424);
#82=VECTOR('',#525,3.);
#83=VECTOR('',#528,3.);
#84=VECTOR('',#529,42.5163970020424);
#85=VECTOR('',#534,50.);
#86=VECTOR('',#537,50.);
#87=VECTOR('',#540,8.50510257216822);
#88=VECTOR('',#541,50.);
#89=VECTOR('',#542,8.50510257216822);
#90=VECTOR('',#545,10.);
#91=VECTOR('',#546,50.);
#92=VECTOR('',#547,10.);
#93=VECTOR('',#550,8.50510257216822);
#94=VECTOR('',#551,8.50510257216822);
#101=FACE_BOUND('',#153,.T.);
#111=FACE_OUTER_BOUND('',#139,.T.);
#112=FACE_OUTER_BOUND('',#140,.T.);
#113=FACE_OUTER_BOUND('',#141,.T.);
#114=FACE_OUTER_BOUND('',#142,.T.);
#115=FACE_OUTER_BOUND('',#143,.T.);
#116=FACE_OUTER_BOUND('',#144,.T.);
#117=FACE_OUTER_BOUND('',#145,.T.);
#118=FACE_OUTER_BOUND('',#146,.T.);
#119=FACE_OUTER_BOUND('',#147,.T.);
#120=FACE_OUTER_BOUND('',#148,.T.);
#121=FACE_OUTER_BOUND('',#149,.T.);
#122=FACE_OUTER_BOUND('',#150,.T.);
#123=FACE_OUTER_BOUND('',#151,.T.);
#124=FACE_OUTER_BOUND('',#152,.T.);
#125=FACE_OUTER_BOUND('',#154,.T.);
#139=EDGE_LOOP('',(#281,#282,#283,#284,#285,#286,#287,#288));
#140=EDGE_LOOP('',(#289,#290,#291,#292,#293,#294,#295,#296));
#141=EDGE_LOOP('',(#297));
#142=EDGE_LOOP('',(#298,#299,#300,#301));
#143=EDGE_LOOP('',(#302,#303,#304,#305));
#144=EDGE_LOOP('',(#306,#307,#308,#309));
#145=EDGE_LOOP('',(#310,#311,#312,#313,#314,#315,#316));
#146=EDGE_LOOP('',(#317,#318,#319,#320,#321,#322,#323));
#147=EDGE_LOOP('',(#324,#325,#326,#327));
#148=EDGE_LOOP('',(#328,#329,#330,#331));
#149=EDGE_LOOP('',(#332,#333,#334,#335));
#150=EDGE_LOOP('',(#336,#337,#338,#339));
#151=EDGE_LOOP('',(#340,#341,#342,#343));
#152=EDGE_LOOP('',(#344,#345,#346,#347));
#153=EDGE_LOOP('',(#348));
#154=EDGE_LOOP('',(#349,#350,#351,#352));
#164=CIRCLE('',#436,7.5);
#165=CIRCLE('',#437,1859.05088195134);
#166=CIRCLE('',#439,7.5);
#167=CIRCLE('',#440,1859.05088195135);
#168=CIRCLE('',#446,25.);
#169=CIRCLE('',#447,25.);
#179=VERTEX_POINT('',#596);
#180=VERTEX_POINT('',#597);
#181=VERTEX_POINT('',#599);
#182=VERTEX_POINT('',#643);
#183=VERTEX_POINT('',#646);
#184=VERTEX_POINT('',#650);
#185=VERTEX_POINT('',#657);
#186=VERTEX_POINT('',#659);
#187=VERTEX_POINT('',#661);
#188=VERTEX_POINT('',#1020);
#189=VERTEX_POINT('',#1022);
#190=VERTEX_POINT('',#1064);
#191=VERTEX_POINT('',#1834);
#192=VERTEX_POINT('',#1841);
#193=VERTEX_POINT('',#1845);
#194=VERTEX_POINT('',#1852);
#195=VERTEX_POINT('',#2824);
#196=VERTEX_POINT('',#2825);
#197=VERTEX_POINT('',#2827);
#198=VERTEX_POINT('',#2829);
#199=VERTEX_POINT('',#2833);
#200=VERTEX_POINT('',#2835);
#201=VERTEX_POINT('',#2839);
#202=VERTEX_POINT('',#2841);
#217=EDGE_CURVE('',#179,#180,#54,.T.);
#218=EDGE_CURVE('',#181,#179,#28,.T.);
#219=EDGE_CURVE('',#181,#182,#55,.T.);
#220=EDGE_CURVE('',#182,#182,#164,.T.);
#221=EDGE_CURVE('',#183,#181,#29,.T.);
#222=EDGE_CURVE('',#183,#184,#165,.T.);
#223=EDGE_CURVE('',#184,#180,#22,.T.);
#224=EDGE_CURVE('',#185,#185,#166,.T.);
#225=EDGE_CURVE('',#185,#186,#56,.T.);
#226=EDGE_CURVE('',#186,#187,#23,.T.);
#227=EDGE_CURVE('',#187,#188,#167,.T.);
#228=EDGE_CURVE('',#189,#188,#30,.T.);
#229=EDGE_CURVE('',#189,#190,#57,.T.);
#230=EDGE_CURVE('',#190,#186,#24,.T.);
#231=EDGE_CURVE('',#179,#189,#31,.T.);
#232=EDGE_CURVE('',#180,#190,#25,.T.);
#233=EDGE_CURVE('',#184,#191,#26,.T.);
#234=EDGE_CURVE('',#192,#183,#58,.T.);
#235=EDGE_CURVE('',#191,#192,#59,.T.);
#236=EDGE_CURVE('',#193,#187,#27,.T.);
#237=EDGE_CURVE('',#194,#193,#60,.T.);
#238=EDGE_CURVE('',#188,#194,#61,.T.);
#239=EDGE_CURVE('',#191,#193,#32,.T.);
#240=EDGE_CURVE('',#192,#194,#33,.T.);
#241=EDGE_CURVE('',#195,#196,#168,.T.);
#242=EDGE_CURVE('',#197,#196,#62,.T.);
#243=EDGE_CURVE('',#198,#197,#169,.T.);
#244=EDGE_CURVE('',#198,#195,#63,.T.);
#245=EDGE_CURVE('',#196,#199,#64,.T.);
#246=EDGE_CURVE('',#200,#199,#65,.T.);
#247=EDGE_CURVE('',#197,#200,#66,.T.);
#248=EDGE_CURVE('',#199,#201,#67,.T.);
#249=EDGE_CURVE('',#202,#201,#68,.T.);
#250=EDGE_CURVE('',#200,#202,#69,.T.);
#251=EDGE_CURVE('',#201,#195,#70,.T.);
#252=EDGE_CURVE('',#202,#198,#71,.T.);
#281=ORIENTED_EDGE('',*,*,#217,.F.);
#282=ORIENTED_EDGE('',*,*,#218,.F.);
#283=ORIENTED_EDGE('',*,*,#219,.T.);
#284=ORIENTED_EDGE('',*,*,#220,.F.);
#285=ORIENTED_EDGE('',*,*,#219,.F.);
#286=ORIENTED_EDGE('',*,*,#221,.F.);
#287=ORIENTED_EDGE('',*,*,#222,.T.);
#288=ORIENTED_EDGE('',*,*,#223,.T.);
#289=ORIENTED_EDGE('',*,*,#224,.T.);
#290=ORIENTED_EDGE('',*,*,#225,.T.);
#291=ORIENTED_EDGE('',*,*,#226,.T.);
#292=ORIENTED_EDGE('',*,*,#227,.T.);
#293=ORIENTED_EDGE('',*,*,#228,.F.);
#294=ORIENTED_EDGE('',*,*,#229,.T.);
#295=ORIENTED_EDGE('',*,*,#230,.T.);
#296=ORIENTED_EDGE('',*,*,#225,.F.);
#297=ORIENTED_EDGE('',*,*,#220,.T.);
#298=ORIENTED_EDGE('',*,*,#229,.F.);
#299=ORIENTED_EDGE('',*,*,#231,.F.);
#300=ORIENTED_EDGE('',*,*,#217,.T.);
#301=ORIENTED_EDGE('',*,*,#232,.T.);
#302=ORIENTED_EDGE('',*,*,#233,.F.);
#303=ORIENTED_EDGE('',*,*,#222,.F.);
#304=ORIENTED_EDGE('',*,*,#234,.F.);
#305=ORIENTED_EDGE('',*,*,#235,.F.);
#306=ORIENTED_EDGE('',*,*,#236,.F.);
#307=ORIENTED_EDGE('',*,*,#237,.F.);
#308=ORIENTED_EDGE('',*,*,#238,.F.);
#309=ORIENTED_EDGE('',*,*,#227,.F.);
#310=ORIENTED_EDGE('',*,*,#233,.T.);
#311=ORIENTED_EDGE('',*,*,#239,.T.);
#312=ORIENTED_EDGE('',*,*,#236,.T.);
#313=ORIENTED_EDGE('',*,*,#226,.F.);
#314=ORIENTED_EDGE('',*,*,#230,.F.);
#315=ORIENTED_EDGE('',*,*,#232,.F.);
#316=ORIENTED_EDGE('',*,*,#223,.F.);
#317=ORIENTED_EDGE('',*,*,#234,.T.);
#318=ORIENTED_EDGE('',*,*,#221,.T.);
#319=ORIENTED_EDGE('',*,*,#218,.T.);
#320=ORIENTED_EDGE('',*,*,#231,.T.);
#321=ORIENTED_EDGE('',*,*,#228,.T.);
#322=ORIENTED_EDGE('',*,*,#238,.T.);
#323=ORIENTED_EDGE('',*,*,#240,.F.);
#324=ORIENTED_EDGE('',*,*,#235,.T.);
#325=ORIENTED_EDGE('',*,*,#240,.T.);
#326=ORIENTED_EDGE('',*,*,#237,.T.);
#327=ORIENTED_EDGE('',*,*,#239,.F.);
#328=ORIENTED_EDGE('',*,*,#241,.T.);
#329=ORIENTED_EDGE('',*,*,#242,.F.);
#330=ORIENTED_EDGE('',*,*,#243,.F.);
#331=ORIENTED_EDGE('',*,*,#244,.T.);
#332=ORIENTED_EDGE('',*,*,#245,.T.);
#333=ORIENTED_EDGE('',*,*,#246,.F.);
#334=ORIENTED_EDGE('',*,*,#247,.F.);
#335=ORIENTED_EDGE('',*,*,#242,.T.);
#336=ORIENTED_EDGE('',*,*,#248,.T.);
#337=ORIENTED_EDGE('',*,*,#249,.F.);
#338=ORIENTED_EDGE('',*,*,#250,.F.);
#339=ORIENTED_EDGE('',*,*,#246,.T.);
#340=ORIENTED_EDGE('',*,*,#251,.T.);
#341=ORIENTED_EDGE('',*,*,#244,.F.);
#342=ORIENTED_EDGE('',*,*,#252,.F.);
#343=ORIENTED_EDGE('',*,*,#249,.T.);
#344=ORIENTED_EDGE('',*,*,#243,.T.);
#345=ORIENTED_EDGE('',*,*,#247,.T.);
#346=ORIENTED_EDGE('',*,*,#250,.T.);
#347=ORIENTED_EDGE('',*,*,#252,.T.);
#348=ORIENTED_EDGE('',*,*,#224,.F.);
#349=ORIENTED_EDGE('',*,*,#241,.F.);
#350=ORIENTED_EDGE('',*,*,#251,.F.);
#351=ORIENTED_EDGE('',*,*,#248,.F.);
#352=ORIENTED_EDGE('',*,*,#245,.F.);
#357=PLANE('',#441);
#358=PLANE('',#443);
#359=PLANE('',#444);
#360=PLANE('',#448);
#361=PLANE('',#449);
#362=PLANE('',#450);
#363=PLANE('',#451);
#364=PLANE('',#452);
#374=ADVANCED_FACE('',(#111),#45,.T.);
#375=ADVANCED_FACE('',(#112),#46,.T.);
#376=ADVANCED_FACE('',(#113),#357,.T.);
#377=ADVANCED_FACE('',(#114),#47,.T.);
#378=ADVANCED_FACE('',(#115),#358,.F.);
#379=ADVANCED_FACE('',(#116),#359,.F.);
#380=ADVANCED_FACE('',(#117),#19,.T.);
#381=ADVANCED_FACE('',(#118),#20,.T.);
#382=ADVANCED_FACE('',(#119),#21,.T.);
#383=ADVANCED_FACE('',(#120),#48,.T.);
#384=ADVANCED_FACE('',(#121),#360,.F.);
#385=ADVANCED_FACE('',(#122),#361,.F.);
#386=ADVANCED_FACE('',(#123),#362,.F.);
#387=ADVANCED_FACE('',(#124,#101),#363,.T.);
#388=ADVANCED_FACE('',(#125),#364,.F.);
#390=CLOSED_SHELL('',(#374,#375,#376,#377,#378,#379,#380,#381,#382,#383,
#384,#385,#386,#387,#388));
#434=AXIS2_PLACEMENT_3D('',#594,#500,#501);
#435=AXIS2_PLACEMENT_3D('',#595,#502,#503);
#436=AXIS2_PLACEMENT_3D('',#645,#506,#507);
#437=AXIS2_PLACEMENT_3D('',#651,#508,#509);
#438=AXIS2_PLACEMENT_3D('',#656,#510,#511);
#439=AXIS2_PLACEMENT_3D('',#658,#512,#513);
#440=AXIS2_PLACEMENT_3D('',#1021,#515,#516);
#441=AXIS2_PLACEMENT_3D('',#1427,#518,#519);
#442=AXIS2_PLACEMENT_3D('',#1428,#520,#521);
#443=AXIS2_PLACEMENT_3D('',#1833,#522,#523);
#444=AXIS2_PLACEMENT_3D('',#1844,#526,#527);
#445=AXIS2_PLACEMENT_3D('',#2823,#530,#531);
#446=AXIS2_PLACEMENT_3D('',#2826,#532,#533);
#447=AXIS2_PLACEMENT_3D('',#2830,#535,#536);
#448=AXIS2_PLACEMENT_3D('',#2832,#538,#539);
#449=AXIS2_PLACEMENT_3D('',#2838,#543,#544);
#450=AXIS2_PLACEMENT_3D('',#2844,#548,#549);
#451=AXIS2_PLACEMENT_3D('',#2847,#552,#553);
#452=AXIS2_PLACEMENT_3D('',#2848,#554,#555);
#500=DIRECTION('axis',(0.,0.,1.));
#501=DIRECTION('refdir',(1.,0.,0.));
#502=DIRECTION('center_axis',(0.,-1.,0.));
#503=DIRECTION('ref_axis',(0.,0.,-1.));
#504=DIRECTION('',(0.,1.,0.));
#505=DIRECTION('',(0.,1.,0.));
#506=DIRECTION('center_axis',(0.,1.,0.));
#507=DIRECTION('ref_axis',(-0.715662544779069,0.,-0.698446219833959));
#508=DIRECTION('center_axis',(0.997979715186782,0.0635333619109602,1.57664132857237E-12));
#509=DIRECTION('ref_axis',(0.000102666233862281,-0.00161267745569481,0.999998694364682));
#510=DIRECTION('center_axis',(0.,-1.,0.));
#511=DIRECTION('ref_axis',(0.,0.,-1.));
#512=DIRECTION('center_axis',(0.,1.,0.));
#513=DIRECTION('ref_axis',(0.,0.,1.));
#514=DIRECTION('',(0.,1.,0.));
#515=DIRECTION('center_axis',(-0.997979715186782,-0.0635333619109597,-1.60052983355074E-12));
#516=DIRECTION('ref_axis',(1.40886995536597E-7,-2.21307290245903E-6,0.999999999997541));
#517=DIRECTION('',(0.,1.,0.));
#518=DIRECTION('center_axis',(0.,1.,0.));
#519=DIRECTION('ref_axis',(-0.715662544779069,0.,-0.698446219833959));
#520=DIRECTION('center_axis',(0.,-1.,0.));
#521=DIRECTION('ref_axis',(0.,0.,-1.));
#522=DIRECTION('center_axis',(-0.997979715186782,-0.0635333619109615,0.));
#523=DIRECTION('ref_axis',(0.,0.,1.));
#524=DIRECTION('',(7.77774425693207E-18,0.,-1.));
#525=DIRECTION('',(-0.0635333619109615,0.997979715186782,0.));
#526=DIRECTION('center_axis',(0.997979715186782,0.063533361910961,0.));
#527=DIRECTION('ref_axis',(0.,0.,-1.));
#528=DIRECTION('',(0.0635333619109615,-0.997979715186782,0.));
#529=DIRECTION('',(-7.77774425693207E-18,0.,1.));
#530=DIRECTION('center_axis',(0.,-1.,0.));
#531=DIRECTION('ref_axis',(-3.21624529935327E-16,0.,1.));
#532=DIRECTION('center_axis',(0.,1.,0.));
#533=DIRECTION('ref_axis',(0.,0.,1.));
#534=DIRECTION('',(0.,-1.,0.));
#535=DIRECTION('center_axis',(0.,1.,0.));
#536=DIRECTION('ref_axis',(0.,0.,1.));
#537=DIRECTION('',(0.,-1.,0.));
#538=DIRECTION('center_axis',(-1.,0.,-4.07925350989523E-16));
#539=DIRECTION('ref_axis',(-4.07925350989523E-16,0.,1.));
#540=DIRECTION('',(3.91608336949942E-16,0.,-1.));
#541=DIRECTION('',(0.,-1.,0.));
#542=DIRECTION('',(3.91608336949942E-16,0.,-1.));
#543=DIRECTION('center_axis',(0.,0.,1.));
#544=DIRECTION('ref_axis',(1.,0.,0.));
#545=DIRECTION('',(-1.,0.,0.));
#546=DIRECTION('',(0.,-1.,0.));
#547=DIRECTION('',(-1.,0.,0.));
#548=DIRECTION('center_axis',(1.,0.,-4.07925350989523E-16));
#549=DIRECTION('ref_axis',(-4.07925350989523E-16,0.,-1.));
#550=DIRECTION('',(3.91608336949942E-16,0.,1.));
#551=DIRECTION('',(3.91608336949942E-16,0.,1.));
#552=DIRECTION('center_axis',(0.,1.,0.));
#553=DIRECTION('ref_axis',(0.,0.,1.));
#554=DIRECTION('center_axis',(0.,1.,0.));
#555=DIRECTION('ref_axis',(0.,0.,1.));
#594=CARTESIAN_POINT('',(0.,0.,0.));
#595=CARTESIAN_POINT('Origin',(0.,240.,0.));
#596=CARTESIAN_POINT('',(-1.90241102001116E-16,217.99585953923,7.50000000439337));
#597=CARTESIAN_POINT('',(-4.06843950140785E-7,234.921557632927,7.50242802810186));
#598=CARTESIAN_POINT('',(-9.18485099360515E-16,240.,7.5));
#599=CARTESIAN_POINT('',(-9.18479639923619E-16,237.99585953923,7.50000000439337));
#600=CARTESIAN_POINT('Ctrl Pts',(-9.1847417994869E-16,237.99585953923,7.50000000439337));
#601=CARTESIAN_POINT('Ctrl Pts',(-1.18775172812193,237.495912211348,7.50000000439337));
#602=CARTESIAN_POINT('Ctrl Pts',(-2.317383311169,236.995967593475,7.13300320026677));
#603=CARTESIAN_POINT('Ctrl Pts',(-3.44714003087638,236.495967593475,6.76596574150984));
#604=CARTESIAN_POINT('Ctrl Pts',(-4.40818170865423,235.995967593475,6.06777834873578));
#605=CARTESIAN_POINT('Ctrl Pts',(-5.36922338643209,235.495967593475,5.36959095596173));
#606=CARTESIAN_POINT('Ctrl Pts',(-6.06747656688843,234.995967593475,4.40859707573286));
#607=CARTESIAN_POINT('Ctrl Pts',(-6.76572974734476,234.495967593475,3.447603195504));
#608=CARTESIAN_POINT('Ctrl Pts',(-7.13284454416054,233.995967593475,2.31787160445521));
#609=CARTESIAN_POINT('Ctrl Pts',(-7.49995934097631,233.495967593475,1.18814001340642));
#610=CARTESIAN_POINT('Ctrl Pts',(-7.5,232.995967593475,0.000256710972401669));
#611=CARTESIAN_POINT('Ctrl Pts',(-7.50004065902369,232.495967593475,-1.18762659146162));
#612=CARTESIAN_POINT('Ctrl Pts',(-7.13300320026677,231.995967593475,-2.317383311169));
#613=CARTESIAN_POINT('Ctrl Pts',(-6.76596574150984,231.495967593475,-3.44714003087638));
#614=CARTESIAN_POINT('Ctrl Pts',(-6.06777834873578,230.995967593475,-4.40818170865423));
#615=CARTESIAN_POINT('Ctrl Pts',(-5.36959095596173,230.495967593475,-5.36922338643209));
#616=CARTESIAN_POINT('Ctrl Pts',(-4.40859707573286,229.995967593475,-6.06747656688843));
#617=CARTESIAN_POINT('Ctrl Pts',(-3.447603195504,229.495967593475,-6.76572974734476));
#618=CARTESIAN_POINT('Ctrl Pts',(-2.31787160445521,228.995967593475,-7.13284454416054));
#619=CARTESIAN_POINT('Ctrl Pts',(-1.18814001340642,228.495967593475,-7.49995934097631));
#620=CARTESIAN_POINT('Ctrl Pts',(-0.000256710972402128,227.995967593475,
-7.5));
#621=CARTESIAN_POINT('Ctrl Pts',(1.18762659146162,227.495967593475,-7.50004065902369));
#622=CARTESIAN_POINT('Ctrl Pts',(2.317383311169,226.995967593475,-7.13300320026677));
#623=CARTESIAN_POINT('Ctrl Pts',(3.44714003087638,226.495967593475,-6.76596574150984));
#624=CARTESIAN_POINT('Ctrl Pts',(4.40818170865423,225.995967593475,-6.06777834873578));
#625=CARTESIAN_POINT('Ctrl Pts',(5.36922338643209,225.495967593475,-5.36959095596173));
#626=CARTESIAN_POINT('Ctrl Pts',(6.06747656688843,224.995967593475,-4.40859707573286));
#627=CARTESIAN_POINT('Ctrl Pts',(6.76572974734476,224.495967593475,-3.447603195504));
#628=CARTESIAN_POINT('Ctrl Pts',(7.13284454416054,223.995967593475,-2.31787160445521));
#629=CARTESIAN_POINT('Ctrl Pts',(7.49995934097631,223.495967593475,-1.18814001340642));
#630=CARTESIAN_POINT('Ctrl Pts',(7.5,222.995967593475,-0.000256710972402588));
#631=CARTESIAN_POINT('Ctrl Pts',(7.50004065902369,222.495967593475,1.18762659146162));
#632=CARTESIAN_POINT('Ctrl Pts',(7.13300320026677,221.995967593475,2.317383311169));
#633=CARTESIAN_POINT('Ctrl Pts',(6.76596574150984,221.495967593475,3.44714003087638));
#634=CARTESIAN_POINT('Ctrl Pts',(6.06777834873579,220.995967593475,4.40818170865423));
#635=CARTESIAN_POINT('Ctrl Pts',(5.36959095596173,220.495967593475,5.36922338643209));
#636=CARTESIAN_POINT('Ctrl Pts',(4.40859707573286,219.995967593475,6.06747656688843));
#637=CARTESIAN_POINT('Ctrl Pts',(3.447603195504,219.495967593475,6.76572974734476));
#638=CARTESIAN_POINT('Ctrl Pts',(2.31787160445521,218.995967593475,7.13284454416054));
#639=CARTESIAN_POINT('Ctrl Pts',(1.18814001340643,218.495967593475,7.49995934097631));
#640=CARTESIAN_POINT('Ctrl Pts',(0.00025671097240121,217.995967593475,7.5));
#641=CARTESIAN_POINT('Ctrl Pts',(0.000128355486249734,217.995913566499,
7.50000000439337));
#642=CARTESIAN_POINT('Ctrl Pts',(5.38002895896315E-16,217.99585953923,7.50000000439337));
#643=CARTESIAN_POINT('',(-9.18485099360515E-16,400.,7.5));
#644=CARTESIAN_POINT('',(-9.18485099360515E-16,240.,7.5));
#645=CARTESIAN_POINT('Origin',(0.,400.,3.5527136788005E-14));
#646=CARTESIAN_POINT('',(0.00025671099249169,237.995967593476,7.49999999788428));
#647=CARTESIAN_POINT('Ctrl Pts',(0.00025671097240121,237.995967593475,7.5));
#648=CARTESIAN_POINT('Ctrl Pts',(0.000128355486236195,237.995913566499,
7.50000000439337));
#649=CARTESIAN_POINT('Ctrl Pts',(-9.1847417994869E-16,237.99585953923,7.50000000439337));
#650=CARTESIAN_POINT('',(0.19085679599498,235.002028447937,7.49999995822451));
#651=CARTESIAN_POINT('Origin',(-5.20522648770767E-6,238.000081810591,-1851.55088195117));
#652=CARTESIAN_POINT('Ctrl Pts',(0.190856796705285,235.002028447915,7.5));
#653=CARTESIAN_POINT('Ctrl Pts',(0.127311648028415,234.975281229334,7.50161706980302));
#654=CARTESIAN_POINT('Ctrl Pts',(0.0636823578853783,234.948453397593,7.50242803155527));
#655=CARTESIAN_POINT('Ctrl Pts',(-4.06843934450864E-7,234.921557632927,
7.50242802810186));
#656=CARTESIAN_POINT('Origin',(0.,240.,0.));
#657=CARTESIAN_POINT('',(0.,150.,7.5));
#658=CARTESIAN_POINT('Origin',(0.,150.,0.));
#659=CARTESIAN_POINT('',(-4.0684396522591E-7,194.921557632927,7.50242802810186));
#660=CARTESIAN_POINT('',(-9.18485099360515E-16,240.,7.5));
#661=CARTESIAN_POINT('',(0.190870214476193,175.002034095778,7.4999996458277));
#662=CARTESIAN_POINT('Ctrl Pts',(-4.06843965232862E-7,194.921557632927,
7.50242802810186));
#663=CARTESIAN_POINT('Ctrl Pts',(-0.152090385415712,194.857323985265,7.50242801985428));
#664=CARTESIAN_POINT('Ctrl Pts',(-0.304485788637936,194.792702491972,7.49779895914529));
#665=CARTESIAN_POINT('Ctrl Pts',(-0.456762644214526,194.727870534021,7.48851081348613));
#666=CARTESIAN_POINT('Ctrl Pts',(-0.609070650330248,194.663025313709,7.47922076779598));
#667=CARTESIAN_POINT('Ctrl Pts',(-0.761259533137463,194.597969762789,7.46526968655078));
#668=CARTESIAN_POINT('Ctrl Pts',(-0.91290272043789,194.532885263598,7.44667945730617));
#669=CARTESIAN_POINT('Ctrl Pts',(-1.06450493068591,194.467818351553,7.42809425151703));
#670=CARTESIAN_POINT('Ctrl Pts',(-1.2155612127976,194.402722732839,7.40487246128588));
#671=CARTESIAN_POINT('Ctrl Pts',(-1.36565093134532,194.337780178401,7.37708776215684));
#672=CARTESIAN_POINT('Ctrl Pts',(-1.51579830432436,194.272812677376,7.34929239000474));
#673=CARTESIAN_POINT('Ctrl Pts',(-1.6649778616245,194.207998581557,7.31693074896081));
#674=CARTESIAN_POINT('Ctrl Pts',(-1.81278187771196,194.143517028959,7.28012693438018));
#675=CARTESIAN_POINT('Ctrl Pts',(-1.92135204017681,194.096151789321,7.25309251248746));
#676=CARTESIAN_POINT('Ctrl Pts',(-2.02918025203168,194.04896593395,7.22366229239575));
#677=CARTESIAN_POINT('Ctrl Pts',(-2.13611185762632,194.002028447915,7.19190186588755));
#678=CARTESIAN_POINT('Ctrl Pts',(-2.2816613117044,193.938139708658,7.14867131011455));
#679=CARTESIAN_POINT('Ctrl Pts',(-2.42624566734731,193.87379055128,7.10091475754277));
#680=CARTESIAN_POINT('Ctrl Pts',(-2.56944875671864,193.809155844927,7.04871331545309));
#681=CARTESIAN_POINT('Ctrl Pts',(-2.71813540129491,193.74204613624,6.99451296753858));
#682=CARTESIAN_POINT('Ctrl Pts',(-2.86533230206808,193.674628800623,6.93552054364116));
#683=CARTESIAN_POINT('Ctrl Pts',(-3.01058579312346,193.607105531561,6.87188471229631));
#684=CARTESIAN_POINT('Ctrl Pts',(-3.15046347852857,193.542081286575,6.81060403165537));
#685=CARTESIAN_POINT('Ctrl Pts',(-3.28853853492898,193.476959054234,6.74501779444794));
#686=CARTESIAN_POINT('Ctrl Pts',(-3.42442461876489,193.411920847683,6.67530840839924));
#687=CARTESIAN_POINT('Ctrl Pts',(-3.5602870648691,193.346893954694,6.60561114847646));
#688=CARTESIAN_POINT('Ctrl Pts',(-3.693960843474,193.281951283189,6.53179244342482));
#689=CARTESIAN_POINT('Ctrl Pts',(-3.82508551083643,193.217273190526,6.45407988420021));
#690=CARTESIAN_POINT('Ctrl Pts',(-3.95624536474471,193.152577741872,6.37634647125995));
#691=CARTESIAN_POINT('Ctrl Pts',(-4.0848543388159,193.088147231022,6.2947174573996));
#692=CARTESIAN_POINT('Ctrl Pts',(-4.21058385833655,193.024157275819,6.20946132033724));
#693=CARTESIAN_POINT('Ctrl Pts',(-4.22508868089454,193.016775056041,6.1996257213086));
#694=CARTESIAN_POINT('Ctrl Pts',(-4.23955521930311,193.009398692253,6.18974188939153));
#695=CARTESIAN_POINT('Ctrl Pts',(-4.25398300016701,193.002028447915,6.17981026821526));
#696=CARTESIAN_POINT('Ctrl Pts',(-4.37904978050105,192.938139708658,6.09371831161215));
#697=CARTESIAN_POINT('Ctrl Pts',(-4.50180008775214,192.87379055128,6.00362010807856));
#698=CARTESIAN_POINT('Ctrl Pts',(-4.62186318631576,192.809155844927,5.90972139815641));
#699=CARTESIAN_POINT('Ctrl Pts',(-4.74652375991947,192.74204613624,5.8122271040762));
#700=CARTESIAN_POINT('Ctrl Pts',(-4.86828667005456,192.674628800622,5.71063563105828));
#701=CARTESIAN_POINT('Ctrl Pts',(-4.98676639590067,192.607105531561,5.6052285617595));
#702=CARTESIAN_POINT('Ctrl Pts',(-5.10086120834454,192.542081286575,5.50372258918893));
#703=CARTESIAN_POINT('Ctrl Pts',(-5.21191112857775,192.476959054234,5.39867883198654));
#704=CARTESIAN_POINT('Ctrl Pts',(-5.31960508912721,192.411920847683,5.29039015693365));
#705=CARTESIAN_POINT('Ctrl Pts',(-5.42728031603782,192.346893954693,5.18212031897172));
#706=CARTESIAN_POINT('Ctrl Pts',(-5.53160039987492,192.281951283188,5.07060708921572));
#707=CARTESIAN_POINT('Ctrl Pts',(-5.632292867741,192.217273190525,4.95617830276943));
#708=CARTESIAN_POINT('Ctrl Pts',(-5.73301235584602,192.152577741871,4.84171881002288));
#709=CARTESIAN_POINT('Ctrl Pts',(-5.83010200617219,192.088147231023,4.72434264585674));
#710=CARTESIAN_POINT('Ctrl Pts',(-5.92333228977468,192.02415727582,4.60440668292466));
#711=CARTESIAN_POINT('Ctrl Pts',(-5.93408782853699,192.016775056042,4.59057023570531));
#712=CARTESIAN_POINT('Ctrl Pts',(-5.94479205212731,192.009398692253,4.5766997467359));
#713=CARTESIAN_POINT('Ctrl Pts',(-5.95544464740897,192.002028447915,4.56279578422008));
#714=CARTESIAN_POINT('Ctrl Pts',(-6.04778634614874,191.938139708657,4.44226970733661));
#715=CARTESIAN_POINT('Ctrl Pts',(-6.13668694968295,191.87379055128,4.31864929275364));
#716=CARTESIAN_POINT('Ctrl Pts',(-6.22185744482296,191.809155844926,4.19224477495645));
#717=CARTESIAN_POINT('Ctrl Pts',(-6.31028930194836,191.742046136239,4.0609999554979));
#718=CARTESIAN_POINT('Ctrl Pts',(-6.39469921942917,191.674628800622,3.92675391456802));
#719=CARTESIAN_POINT('Ctrl Pts',(-6.47480755900329,191.60710553156,3.78989358567263));
#720=CARTESIAN_POINT('Ctrl Pts',(-6.55195110329862,191.542081286575,3.65809843300132));
#721=CARTESIAN_POINT('Ctrl Pts',(-6.6251055474419,191.476959054234,3.5238795706418));
#722=CARTESIAN_POINT('Ctrl Pts',(-6.69406554949839,191.411920847682,3.38761165659044));
#723=CARTESIAN_POINT('Ctrl Pts',(-6.76301355578597,191.346893954693,3.2513674466916));
#724=CARTESIAN_POINT('Ctrl Pts',(-6.82776836820671,191.281951283189,3.11307538412042));
#725=CARTESIAN_POINT('Ctrl Pts',(-6.88817215625433,191.217273190527,2.97313145734446));
#726=CARTESIAN_POINT('Ctrl Pts',(-6.94859215330858,191.152577741872,2.83314997742638));
#727=CARTESIAN_POINT('Ctrl Pts',(-7.00465866845448,191.088147231024,2.69151625970926));
#728=CARTESIAN_POINT('Ctrl Pts',(-7.05626368640816,191.024157275821,2.54864063860052));
#729=CARTESIAN_POINT('Ctrl Pts',(-7.06221711430205,191.016775056042,2.53215775104821));
#730=CARTESIAN_POINT('Ctrl Pts',(-7.06811121908795,191.009398692254,2.51565834512789));
#731=CARTESIAN_POINT('Ctrl Pts',(-7.07394587853975,191.002028447915,2.49914305799789));
#732=CARTESIAN_POINT('Ctrl Pts',(-7.12452344682944,190.938139708658,2.35598079299494));
#733=CARTESIAN_POINT('Ctrl Pts',(-7.17087213616523,190.87379055128,2.21093899485705));
#734=CARTESIAN_POINT('Ctrl Pts',(-7.21281294639898,190.809155844927,2.06440202409992));
#735=CARTESIAN_POINT('Ctrl Pts',(-7.2563597607299,190.74204613624,1.91225383662786));
#736=CARTESIAN_POINT('Ctrl Pts',(-7.29515405471514,190.674628800622,1.75849416561916));
#737=CARTESIAN_POINT('Ctrl Pts',(-7.32904944559233,190.607105531561,1.60357741968119));
#738=CARTESIAN_POINT('Ctrl Pts',(-7.36169037413291,190.542081286575,1.45439411472324));
#739=CARTESIAN_POINT('Ctrl Pts',(-7.38978847549664,190.476959054234,1.30413842461194));
#740=CARTESIAN_POINT('Ctrl Pts',(-7.41326423358634,190.411920847683,1.15323012442364));
#741=CARTESIAN_POINT('Ctrl Pts',(-7.43673590800807,190.346893954693,1.00234807511892));
#742=CARTESIAN_POINT('Ctrl Pts',(-7.45558679680081,190.281951283188,0.850814170351292));
#743=CARTESIAN_POINT('Ctrl Pts',(-7.46978916139915,190.217273190524,0.69905378984192));
#744=CARTESIAN_POINT('Ctrl Pts',(-7.48399533711969,190.15257774187,0.547252685314279));
#745=CARTESIAN_POINT('Ctrl Pts',(-7.493550535944,190.088147231021,0.395225509155809));
#746=CARTESIAN_POINT('Ctrl Pts',(-7.49847882953778,190.024157275818,0.243395891136868));
#747=CARTESIAN_POINT('Ctrl Pts',(-7.49904738356042,190.01677505604,0.225880023131504));
#748=CARTESIAN_POINT('Ctrl Pts',(-7.49955441349822,190.009398692253,0.208366777073135));
#749=CARTESIAN_POINT('Ctrl Pts',(-7.5,190.002028447915,0.190856796705286));
#750=CARTESIAN_POINT('Ctrl Pts',(-7.50386255306115,189.938139708658,0.0390720635508336));
#751=CARTESIAN_POINT('Ctrl Pts',(-7.50312239555638,189.87379055128,-0.113193416375283));
#752=CARTESIAN_POINT('Ctrl Pts',(-7.4977280621597,189.809155844927,-0.265518780412243));
#753=CARTESIAN_POINT('Ctrl Pts',(-7.49212716810079,189.74204613624,-0.423677011229148));
#754=CARTESIAN_POINT('Ctrl Pts',(-7.48150838279932,189.674628800622,-0.581899244411572));
#755=CARTESIAN_POINT('Ctrl Pts',(-7.46587290795734,189.60710553156,-0.739708076931111));
#756=CARTESIAN_POINT('Ctrl Pts',(-7.45081609923473,189.542081286575,-0.891676432865303));
#757=CARTESIAN_POINT('Ctrl Pts',(-7.43110741988625,189.476959054234,-1.04326087688739));
#758=CARTESIAN_POINT('Ctrl Pts',(-7.40680096324194,189.411920847682,-1.19403760735031));
#759=CARTESIAN_POINT('Ctrl Pts',(-7.38249873476802,189.346893954693,-1.3447881098148));
#760=CARTESIAN_POINT('Ctrl Pts',(-7.35360044359543,189.281951283189,-1.49473066237826));
#761=CARTESIAN_POINT('Ctrl Pts',(-7.32021115834367,189.217273190526,-1.64345213319688));
#762=CARTESIAN_POINT('Ctrl Pts',(-7.28681291327052,189.152577741871,-1.79221351256119));
#763=CARTESIAN_POINT('Ctrl Pts',(-7.24892146633721,189.088147231023,-1.93975266792177));
#764=CARTESIAN_POINT('Ctrl Pts',(-7.20669061985663,189.02415727582,-2.08567414197882));
#765=CARTESIAN_POINT('Ctrl Pts',(-7.20181864597947,189.016775056041,-2.10250841524041));
#766=CARTESIAN_POINT('Ctrl Pts',(-7.19688896944668,189.009398692253,-2.11932118289446));
#767=CARTESIAN_POINT('Ctrl Pts',(-7.19190186588755,189.002028447915,-2.13611185762632));
#768=CARTESIAN_POINT('Ctrl Pts',(-7.14867131011472,188.938139708658,-2.28166131170383));
#769=CARTESIAN_POINT('Ctrl Pts',(-7.10091475754315,188.873790551281,-2.42624566734616));
#770=CARTESIAN_POINT('Ctrl Pts',(-7.0487133154537,188.809155844928,-2.56944875671694));
#771=CARTESIAN_POINT('Ctrl Pts',(-6.99451296753918,188.742046136241,-2.71813540129337));
#772=CARTESIAN_POINT('Ctrl Pts',(-6.93552054364173,188.674628800623,-2.8653323020667));
#773=CARTESIAN_POINT('Ctrl Pts',(-6.87188471229685,188.607105531561,-3.01058579312224));
#774=CARTESIAN_POINT('Ctrl Pts',(-6.81060403165581,188.542081286576,-3.15046347852764));
#775=CARTESIAN_POINT('Ctrl Pts',(-6.74501779444825,188.476959054235,-3.28853853492835));
#776=CARTESIAN_POINT('Ctrl Pts',(-6.67530840839942,188.411920847683,-3.42442461876454));
#777=CARTESIAN_POINT('Ctrl Pts',(-6.60561114847652,188.346893954694,-3.560287064869));
#778=CARTESIAN_POINT('Ctrl Pts',(-6.53179244342476,188.281951283189,-3.69396084347412));
#779=CARTESIAN_POINT('Ctrl Pts',(-6.4540798842,188.217273190526,-3.82508551083678));
#780=CARTESIAN_POINT('Ctrl Pts',(-6.37634647125945,188.152577741871,-3.95624536474554));
#781=CARTESIAN_POINT('Ctrl Pts',(-6.29471745739878,188.088147231022,-4.08485433881718));
#782=CARTESIAN_POINT('Ctrl Pts',(-6.20946132033607,188.024157275818,-4.21058385833828));
#783=CARTESIAN_POINT('Ctrl Pts',(-6.19962572130782,188.01677505604,-4.22508868089568));
#784=CARTESIAN_POINT('Ctrl Pts',(-6.18974188939115,188.009398692253,-4.23955521930367));
#785=CARTESIAN_POINT('Ctrl Pts',(-6.17981026821527,188.002028447915,-4.25398300016699));
#786=CARTESIAN_POINT('Ctrl Pts',(-6.09371831161279,187.938139708658,-4.37904978050011));
#787=CARTESIAN_POINT('Ctrl Pts',(-6.00362010807988,187.873790551281,-4.50180008775034));
#788=CARTESIAN_POINT('Ctrl Pts',(-5.90972139815848,187.809155844928,-4.62186318631311));
#789=CARTESIAN_POINT('Ctrl Pts',(-5.81222710407815,187.742046136241,-4.74652375991708));
#790=CARTESIAN_POINT('Ctrl Pts',(-5.71063563106011,187.674628800624,-4.86828667005243));
#791=CARTESIAN_POINT('Ctrl Pts',(-5.60522856176118,187.607105531562,-4.98676639589878));
#792=CARTESIAN_POINT('Ctrl Pts',(-5.50372258919049,187.542081286576,-5.10086120834287));
#793=CARTESIAN_POINT('Ctrl Pts',(-5.39867883198795,187.476959054235,-5.21191112857629));
#794=CARTESIAN_POINT('Ctrl Pts',(-5.29039015693491,187.411920847684,-5.31960508912596));
#795=CARTESIAN_POINT('Ctrl Pts',(-5.18212031897362,187.346893954694,-5.42728031603598));
#796=CARTESIAN_POINT('Ctrl Pts',(-5.07060708921829,187.28195128319,-5.53160039987254));
#797=CARTESIAN_POINT('Ctrl Pts',(-4.9561783027727,187.217273190527,-5.63229286773812));
#798=CARTESIAN_POINT('Ctrl Pts',(-4.84171881002545,187.152577741872,-5.73301235584388));
#799=CARTESIAN_POINT('Ctrl Pts',(-4.72434264585857,187.088147231023,-5.83010200617073));
#800=CARTESIAN_POINT('Ctrl Pts',(-4.60440668292569,187.024157275821,-5.92333228977387));
#801=CARTESIAN_POINT('Ctrl Pts',(-4.59057023570601,187.016775056042,-5.93408782853645));
#802=CARTESIAN_POINT('Ctrl Pts',(-4.57669974673625,187.009398692254,-5.94479205212704));
#803=CARTESIAN_POINT('Ctrl Pts',(-4.56279578422009,187.002028447915,-5.95544464740895));
#804=CARTESIAN_POINT('Ctrl Pts',(-4.44226970733713,186.938139708658,-6.04778634614834));
#805=CARTESIAN_POINT('Ctrl Pts',(-4.31864929275469,186.87379055128,-6.1366869496822));
#806=CARTESIAN_POINT('Ctrl Pts',(-4.19224477495805,186.809155844927,-6.22185744482188));
#807=CARTESIAN_POINT('Ctrl Pts',(-4.0609999554994,186.74204613624,-6.31028930194741));
#808=CARTESIAN_POINT('Ctrl Pts',(-3.9267539145694,186.674628800622,-6.39469921942832));
#809=CARTESIAN_POINT('Ctrl Pts',(-3.78989358567389,186.607105531561,-6.47480755900255));
#810=CARTESIAN_POINT('Ctrl Pts',(-3.65809843300279,186.542081286575,-6.55195110329779));
#811=CARTESIAN_POINT('Ctrl Pts',(-3.52387957064348,186.476959054235,-6.62510554744101));
#812=CARTESIAN_POINT('Ctrl Pts',(-3.38761165659234,186.411920847683,-6.69406554949743));
#813=CARTESIAN_POINT('Ctrl Pts',(-3.25136744669377,186.346893954695,-6.76301355578491));
#814=CARTESIAN_POINT('Ctrl Pts',(-3.11307538412286,186.28195128319,-6.82776836820559));
#815=CARTESIAN_POINT('Ctrl Pts',(-2.97313145734719,186.217273190528,-6.88817215625315));
#816=CARTESIAN_POINT('Ctrl Pts',(-2.83314997742771,186.152577741873,-6.94859215330807));
#817=CARTESIAN_POINT('Ctrl Pts',(-2.69151625970919,186.088147231024,-7.00465866845454));
#818=CARTESIAN_POINT('Ctrl Pts',(-2.54864063859899,186.024157275821,-7.05626368640871));
#819=CARTESIAN_POINT('Ctrl Pts',(-2.53215775104719,186.016775056042,-7.06221711430242));
#820=CARTESIAN_POINT('Ctrl Pts',(-2.51565834512738,186.009398692254,-7.06811121908813));
#821=CARTESIAN_POINT('Ctrl Pts',(-2.49914305799789,186.002028447915,-7.07394587853975));
#822=CARTESIAN_POINT('Ctrl Pts',(-2.35598079299478,185.938139708658,-7.12452344682949));
#823=CARTESIAN_POINT('Ctrl Pts',(-2.21093899485675,185.87379055128,-7.17087213616532));
#824=CARTESIAN_POINT('Ctrl Pts',(-2.06440202409945,185.809155844927,-7.21281294639912));
#825=CARTESIAN_POINT('Ctrl Pts',(-1.91225383662743,185.74204613624,-7.25635976073001));
#826=CARTESIAN_POINT('Ctrl Pts',(-1.75849416561874,185.674628800622,-7.29515405471524));
#827=CARTESIAN_POINT('Ctrl Pts',(-1.60357741968081,185.60710553156,-7.32904944559241));
#828=CARTESIAN_POINT('Ctrl Pts',(-1.45439411472211,185.542081286575,-7.36169037413315));
#829=CARTESIAN_POINT('Ctrl Pts',(-1.30413842461007,185.476959054234,-7.38978847549698));
#830=CARTESIAN_POINT('Ctrl Pts',(-1.15323012442101,185.411920847682,-7.41326423358675));
#831=CARTESIAN_POINT('Ctrl Pts',(-1.002348075116,185.346893954692,-7.43673590800846));
#832=CARTESIAN_POINT('Ctrl Pts',(-0.850814170348105,185.281951283187,-7.45558679680118));
#833=CARTESIAN_POINT('Ctrl Pts',(-0.699053789838449,185.217273190523,-7.46978916139948));
#834=CARTESIAN_POINT('Ctrl Pts',(-0.547252685310788,185.152577741868,-7.48399533711995));
#835=CARTESIAN_POINT('Ctrl Pts',(-0.395225509152289,185.088147231019,-7.49355053594419));
#836=CARTESIAN_POINT('Ctrl Pts',(-0.243395891133334,185.024157275817,-7.4984788295379));
#837=CARTESIAN_POINT('Ctrl Pts',(-0.225880023129145,185.016775056039,-7.49904738356049));
#838=CARTESIAN_POINT('Ctrl Pts',(-0.208366777071962,185.009398692252,-7.49955441349825));
#839=CARTESIAN_POINT('Ctrl Pts',(-0.190856796705286,185.002028447915,-7.5));
#840=CARTESIAN_POINT('Ctrl Pts',(-0.0390720635516772,184.938139708658,-7.50386255306113));
#841=CARTESIAN_POINT('Ctrl Pts',(0.113193416373591,184.873790551281,-7.50312239555639));
#842=CARTESIAN_POINT('Ctrl Pts',(0.265518780409704,184.809155844928,-7.49772806215979));
#843=CARTESIAN_POINT('Ctrl Pts',(0.42367701122682,184.742046136241,-7.49212716810092));
#844=CARTESIAN_POINT('Ctrl Pts',(0.581899244409438,184.674628800623,-7.48150838279949));
#845=CARTESIAN_POINT('Ctrl Pts',(0.739708076929191,184.607105531561,-7.46587290795754));
#846=CARTESIAN_POINT('Ctrl Pts',(0.891676432862843,184.542081286576,-7.45081609923501));
#847=CARTESIAN_POINT('Ctrl Pts',(1.04326087688443,184.476959054235,-7.43110741988665));
#848=CARTESIAN_POINT('Ctrl Pts',(1.19403760734682,184.411920847684,-7.4068009632425));
#849=CARTESIAN_POINT('Ctrl Pts',(1.34478810981303,184.346893954694,-7.38249873476838));
#850=CARTESIAN_POINT('Ctrl Pts',(1.49473066237817,184.281951283189,-7.35360044359548));
#851=CARTESIAN_POINT('Ctrl Pts',(1.64345213319847,184.217273190525,-7.32021115834331));
#852=CARTESIAN_POINT('Ctrl Pts',(1.79221351256205,184.152577741871,-7.28681291327029));
#853=CARTESIAN_POINT('Ctrl Pts',(1.93975266792193,184.088147231022,-7.24892146633715));
#854=CARTESIAN_POINT('Ctrl Pts',(2.08567414197828,184.02415727582,-7.20669061985679));
#855=CARTESIAN_POINT('Ctrl Pts',(2.10250841524006,184.016775056042,-7.20181864597957));
#856=CARTESIAN_POINT('Ctrl Pts',(2.11932118289428,184.009398692253,-7.19688896944673));
#857=CARTESIAN_POINT('Ctrl Pts',(2.13611185762632,184.002028447915,-7.19190186588755));
#858=CARTESIAN_POINT('Ctrl Pts',(2.28166131170458,183.938139708658,-7.14867131011449));
#859=CARTESIAN_POINT('Ctrl Pts',(2.42624566734765,183.87379055128,-7.10091475754266));
#860=CARTESIAN_POINT('Ctrl Pts',(2.56944875671915,183.809155844927,-7.0487133154529));
#861=CARTESIAN_POINT('Ctrl Pts',(2.71813540129538,183.74204613624,-6.9945129675384));
#862=CARTESIAN_POINT('Ctrl Pts',(2.86533230206852,183.674628800622,-6.93552054364098));
#863=CARTESIAN_POINT('Ctrl Pts',(3.01058579312386,183.60710553156,-6.87188471229614));
#864=CARTESIAN_POINT('Ctrl Pts',(3.15046347852959,183.542081286575,-6.81060403165491));
#865=CARTESIAN_POINT('Ctrl Pts',(3.28853853493061,183.476959054234,-6.74501779444716));
#866=CARTESIAN_POINT('Ctrl Pts',(3.4244246187671,183.411920847682,-6.6753084083981));
#867=CARTESIAN_POINT('Ctrl Pts',(3.5602870648721,183.346893954692,-6.60561114847487));
#868=CARTESIAN_POINT('Ctrl Pts',(3.69396084347772,183.281951283188,-6.53179244342274));
#869=CARTESIAN_POINT('Ctrl Pts',(3.82508551084086,183.217273190524,-6.45407988419758));
#870=CARTESIAN_POINT('Ctrl Pts',(3.95624536474775,183.15257774187,-6.37634647125802));
#871=CARTESIAN_POINT('Ctrl Pts',(4.08485433881761,183.088147231021,-6.29471745739845));
#872=CARTESIAN_POINT('Ctrl Pts',(4.21058385833698,183.024157275819,-6.20946132033695));
#873=CARTESIAN_POINT('Ctrl Pts',(4.22508868089482,183.016775056041,-6.19962572130841));
#874=CARTESIAN_POINT('Ctrl Pts',(4.23955521930325,183.009398692253,-6.18974188939143));
#875=CARTESIAN_POINT('Ctrl Pts',(4.25398300016701,183.002028447915,-6.17981026821526));
#876=CARTESIAN_POINT('Ctrl Pts',(4.37904978050103,182.938139708658,-6.09371831161216));
#877=CARTESIAN_POINT('Ctrl Pts',(4.50180008775213,182.87379055128,-6.00362010807857));
#878=CARTESIAN_POINT('Ctrl Pts',(4.62186318631574,182.809155844927,-5.90972139815642));
#879=CARTESIAN_POINT('Ctrl Pts',(4.74652375991945,182.74204613624,-5.81222710407621));
#880=CARTESIAN_POINT('Ctrl Pts',(4.86828667005454,182.674628800622,-5.7106356310583));
#881=CARTESIAN_POINT('Ctrl Pts',(4.98676639590065,182.607105531561,-5.60522856175951));
#882=CARTESIAN_POINT('Ctrl Pts',(5.10086120834469,182.542081286575,-5.5037225891888));
#883=CARTESIAN_POINT('Ctrl Pts',(5.21191112857806,182.476959054234,-5.39867883198624));
#884=CARTESIAN_POINT('Ctrl Pts',(5.31960508912767,182.411920847683,-5.29039015693319));
#885=CARTESIAN_POINT('Ctrl Pts',(5.42728031603767,182.346893954693,-5.18212031897185));
#886=CARTESIAN_POINT('Ctrl Pts',(5.53160039987421,182.281951283189,-5.07060708921647));
#887=CARTESIAN_POINT('Ctrl Pts',(5.63229286773977,182.217273190526,-4.95617830277083));
#888=CARTESIAN_POINT('Ctrl Pts',(5.73301235584584,182.152577741871,-4.84171881002315));
#889=CARTESIAN_POINT('Ctrl Pts',(5.83010200617298,182.088147231022,-4.72434264585582));
#890=CARTESIAN_POINT('Ctrl Pts',(5.92333228977637,182.024157275819,-4.60440668292248));
#891=CARTESIAN_POINT('Ctrl Pts',(5.9340878285381,182.016775056041,-4.59057023570386));
#892=CARTESIAN_POINT('Ctrl Pts',(5.94479205212786,182.009398692253,-4.57669974673518));
#893=CARTESIAN_POINT('Ctrl Pts',(5.95544464740895,182.002028447915,-4.56279578422009));
#894=CARTESIAN_POINT('Ctrl Pts',(6.04778634614845,181.938139708658,-4.442269707337));
#895=CARTESIAN_POINT('Ctrl Pts',(6.1366869496824,181.87379055128,-4.3186492927544));
#896=CARTESIAN_POINT('Ctrl Pts',(6.22185744482218,181.809155844927,-4.19224477495761));
#897=CARTESIAN_POINT('Ctrl Pts',(6.31028930194767,181.74204613624,-4.06099995549899));
#898=CARTESIAN_POINT('Ctrl Pts',(6.39469921942856,181.674628800622,-3.92675391456902));
#899=CARTESIAN_POINT('Ctrl Pts',(6.47480755900275,181.60710553156,-3.78989358567354));
#900=CARTESIAN_POINT('Ctrl Pts',(6.5519511032983,181.542081286575,-3.65809843300192));
#901=CARTESIAN_POINT('Ctrl Pts',(6.62510554744178,181.476959054234,-3.52387957064205));
#902=CARTESIAN_POINT('Ctrl Pts',(6.69406554949843,181.411920847682,-3.38761165659035));
#903=CARTESIAN_POINT('Ctrl Pts',(6.76301355578636,181.346893954693,-3.25136744669082));
#904=CARTESIAN_POINT('Ctrl Pts',(6.8277683682074,181.281951283189,-3.11307538411894));
#905=CARTESIAN_POINT('Ctrl Pts',(6.88817215625527,181.217273190526,-2.97313145734227));
#906=CARTESIAN_POINT('Ctrl Pts',(6.94859215331014,181.152577741871,-2.83314997742263));
#907=CARTESIAN_POINT('Ctrl Pts',(7.00465866845655,181.088147231021,-2.69151625970395));
#908=CARTESIAN_POINT('Ctrl Pts',(7.05626368641066,181.024157275818,-2.54864063859361));
#909=CARTESIAN_POINT('Ctrl Pts',(7.0622171143037,181.01677505604,-2.5321577510436));
#910=CARTESIAN_POINT('Ctrl Pts',(7.06811121908876,181.009398692253,-2.51565834512559));
#911=CARTESIAN_POINT('Ctrl Pts',(7.07394587853975,181.002028447915,-2.4991430579979));
#912=CARTESIAN_POINT('Ctrl Pts',(7.12452344682943,180.938139708658,-2.35598079299495));
#913=CARTESIAN_POINT('Ctrl Pts',(7.17087213616523,180.87379055128,-2.21093899485704));
#914=CARTESIAN_POINT('Ctrl Pts',(7.21281294639899,180.809155844927,-2.0644020240999));
#915=CARTESIAN_POINT('Ctrl Pts',(7.2563597607299,180.74204613624,-1.91225383662784));
#916=CARTESIAN_POINT('Ctrl Pts',(7.29515405471515,180.674628800622,-1.75849416561912));
#917=CARTESIAN_POINT('Ctrl Pts',(7.32904944559233,180.607105531561,-1.60357741968115));
#918=CARTESIAN_POINT('Ctrl Pts',(7.36169037413299,180.542081286575,-1.45439411472287));
#919=CARTESIAN_POINT('Ctrl Pts',(7.38978847549676,180.476959054234,-1.30413842461125));
#920=CARTESIAN_POINT('Ctrl Pts',(7.4132642335865,180.411920847682,-1.15323012442261));
#921=CARTESIAN_POINT('Ctrl Pts',(7.43673590800803,180.346893954693,-1.00234807511903));
#922=CARTESIAN_POINT('Ctrl Pts',(7.45558679680064,180.281951283189,-0.850814170352573));
#923=CARTESIAN_POINT('Ctrl Pts',(7.46978916139892,180.217273190526,-0.699053789844363));
#924=CARTESIAN_POINT('Ctrl Pts',(7.48399533711951,180.152577741871,-0.547252685316772));
#925=CARTESIAN_POINT('Ctrl Pts',(7.49355053594387,180.088147231022,-0.39522550915836));
#926=CARTESIAN_POINT('Ctrl Pts',(7.4984788295377,180.024157275819,-0.243395891139465));
#927=CARTESIAN_POINT('Ctrl Pts',(7.49904738356037,180.016775056041,-0.225880023133238));
#928=CARTESIAN_POINT('Ctrl Pts',(7.49955441349819,180.009398692253,-0.208366777073998));
#929=CARTESIAN_POINT('Ctrl Pts',(7.5,180.002028447915,-0.190856796705287));
#930=CARTESIAN_POINT('Ctrl Pts',(7.50386255306115,179.938139708658,-0.0390720635508177));
#931=CARTESIAN_POINT('Ctrl Pts',(7.50312239555638,179.87379055128,0.113193416375312));
#932=CARTESIAN_POINT('Ctrl Pts',(7.49772806215969,179.809155844927,0.265518780412289));
#933=CARTESIAN_POINT('Ctrl Pts',(7.49212716810078,179.74204613624,0.42367701122919));
#934=CARTESIAN_POINT('Ctrl Pts',(7.48150838279932,179.674628800622,0.581899244411606));
#935=CARTESIAN_POINT('Ctrl Pts',(7.46587290795734,179.60710553156,0.739708076931141));
#936=CARTESIAN_POINT('Ctrl Pts',(7.45081609923473,179.542081286575,0.891676432865285));
#937=CARTESIAN_POINT('Ctrl Pts',(7.43110741988625,179.476959054234,1.04326087688732));
#938=CARTESIAN_POINT('Ctrl Pts',(7.40680096324196,179.411920847682,1.1940376073502));
#939=CARTESIAN_POINT('Ctrl Pts',(7.38249873476815,179.346893954694,1.34478810981401));
#940=CARTESIAN_POINT('Ctrl Pts',(7.35360044359571,179.281951283189,1.4947306623768));
#941=CARTESIAN_POINT('Ctrl Pts',(7.32021115834415,179.217273190527,1.64345213319477));
#942=CARTESIAN_POINT('Ctrl Pts',(7.28681291327109,179.152577741872,1.79221351255885));
#943=CARTESIAN_POINT('Ctrl Pts',(7.24892146633789,179.088147231024,1.93975266791923));
#944=CARTESIAN_POINT('Ctrl Pts',(7.20669061985743,179.024157275821,2.08567414197607));
#945=CARTESIAN_POINT('Ctrl Pts',(7.20181864598001,179.016775056042,2.10250841523858));
#946=CARTESIAN_POINT('Ctrl Pts',(7.19688896944695,179.009398692254,2.11932118289354));
#947=CARTESIAN_POINT('Ctrl Pts',(7.19190186588755,179.002028447915,2.13611185762632));
#948=CARTESIAN_POINT('Ctrl Pts',(7.14867131011455,178.938139708658,2.2816613117044));
#949=CARTESIAN_POINT('Ctrl Pts',(7.10091475754278,178.87379055128,2.42624566734728));
#950=CARTESIAN_POINT('Ctrl Pts',(7.0487133154531,178.809155844927,2.56944875671861));
#951=CARTESIAN_POINT('Ctrl Pts',(6.99451296753859,178.74204613624,2.71813540129489));
#952=CARTESIAN_POINT('Ctrl Pts',(6.93552054364116,178.674628800623,2.86533230206808));
#953=CARTESIAN_POINT('Ctrl Pts',(6.87188471229631,178.607105531561,3.01058579312346));
#954=CARTESIAN_POINT('Ctrl Pts',(6.81060403165535,178.542081286575,3.15046347852861));
#955=CARTESIAN_POINT('Ctrl Pts',(6.7450177944479,178.476959054234,3.28853853492906));
#956=CARTESIAN_POINT('Ctrl Pts',(6.67530840839917,178.411920847683,3.42442461876501));
#957=CARTESIAN_POINT('Ctrl Pts',(6.60561114847623,178.346893954694,3.56028706486955));
#958=CARTESIAN_POINT('Ctrl Pts',(6.53179244342441,178.281951283189,3.69396084347474));
#959=CARTESIAN_POINT('Ctrl Pts',(6.4540798841996,178.217273190526,3.82508551083747));
#960=CARTESIAN_POINT('Ctrl Pts',(6.37634647126001,178.152577741872,3.95624536474455));
#961=CARTESIAN_POINT('Ctrl Pts',(6.29471745740041,178.088147231023,4.08485433881459));
#962=CARTESIAN_POINT('Ctrl Pts',(6.20946132033887,178.02415727582,4.21058385833414));
#963=CARTESIAN_POINT('Ctrl Pts',(6.1996257213097,178.016775056042,4.22508868089293));
#964=CARTESIAN_POINT('Ctrl Pts',(6.18974188939208,178.009398692254,4.23955521930231));
#965=CARTESIAN_POINT('Ctrl Pts',(6.17981026821526,178.002028447915,4.25398300016701));
#966=CARTESIAN_POINT('Ctrl Pts',(6.09371831161207,177.938139708658,4.37904978050116));
#967=CARTESIAN_POINT('Ctrl Pts',(6.0036201080784,177.87379055128,4.50180008775236));
#968=CARTESIAN_POINT('Ctrl Pts',(5.90972139815616,177.809155844927,4.62186318631608));
#969=CARTESIAN_POINT('Ctrl Pts',(5.81222710407596,177.74204613624,4.74652375991976));
#970=CARTESIAN_POINT('Ctrl Pts',(5.71063563105806,177.674628800622,4.86828667005482));
#971=CARTESIAN_POINT('Ctrl Pts',(5.6052285617593,177.60710553156,4.98676639590089));
#972=CARTESIAN_POINT('Ctrl Pts',(5.5037225891889,177.542081286575,5.10086120834457));
#973=CARTESIAN_POINT('Ctrl Pts',(5.39867883198667,177.476959054235,5.2119111285776));
#974=CARTESIAN_POINT('Ctrl Pts',(5.29039015693398,177.411920847683,5.31960508912689));
#975=CARTESIAN_POINT('Ctrl Pts',(5.18212031897253,177.346893954694,5.42728031603702));
#976=CARTESIAN_POINT('Ctrl Pts',(5.07060708921705,177.281951283189,5.53160039987369));
#977=CARTESIAN_POINT('Ctrl Pts',(4.95617830277129,177.217273190526,5.63229286773936));
#978=CARTESIAN_POINT('Ctrl Pts',(4.84171881002452,177.152577741872,5.73301235584465));
#979=CARTESIAN_POINT('Ctrl Pts',(4.72434264585812,177.088147231023,5.83010200617108));
#980=CARTESIAN_POINT('Ctrl Pts',(4.60440668292578,177.024157275821,5.92333228977381));
#981=CARTESIAN_POINT('Ctrl Pts',(4.59057023570606,177.016775056042,5.93408782853641));
#982=CARTESIAN_POINT('Ctrl Pts',(4.57669974673629,177.009398692254,5.94479205212701));
#983=CARTESIAN_POINT('Ctrl Pts',(4.56279578422009,177.002028447915,5.95544464740895));
#984=CARTESIAN_POINT('Ctrl Pts',(4.44226970733713,176.938139708658,6.04778634614834));
#985=CARTESIAN_POINT('Ctrl Pts',(4.31864929275468,176.87379055128,6.1366869496822));
#986=CARTESIAN_POINT('Ctrl Pts',(4.19224477495804,176.809155844927,6.22185744482189));
#987=CARTESIAN_POINT('Ctrl Pts',(4.06099995549939,176.74204613624,6.31028930194742));
#988=CARTESIAN_POINT('Ctrl Pts',(3.92675391456939,176.674628800622,6.39469921942833));
#989=CARTESIAN_POINT('Ctrl Pts',(3.78989358567388,176.607105531561,6.47480755900255));
#990=CARTESIAN_POINT('Ctrl Pts',(3.65809843300261,176.542081286575,6.5519511032979));
#991=CARTESIAN_POINT('Ctrl Pts',(3.52387957064311,176.476959054234,6.62510554744121));
#992=CARTESIAN_POINT('Ctrl Pts',(3.38761165659179,176.411920847683,6.69406554949771));
#993=CARTESIAN_POINT('Ctrl Pts',(3.25136744669221,176.346893954694,6.76301355578569));
#994=CARTESIAN_POINT('Ctrl Pts',(3.11307538412028,176.281951283189,6.82776836820679));
#995=CARTESIAN_POINT('Ctrl Pts',(2.97313145734355,176.217273190526,6.88817215625472));
#996=CARTESIAN_POINT('Ctrl Pts',(2.83314997742486,176.152577741872,6.94859215330921));
#997=CARTESIAN_POINT('Ctrl Pts',(2.69151625970714,176.088147231023,7.00465866845531));
#998=CARTESIAN_POINT('Ctrl Pts',(2.54864063859777,176.02415727582,7.05626368640916));
#999=CARTESIAN_POINT('Ctrl Pts',(2.53215775104638,176.016775056042,7.06221711430271));
#1000=CARTESIAN_POINT('Ctrl Pts',(2.51565834512697,176.009398692253,7.06811121908827));
#1001=CARTESIAN_POINT('Ctrl Pts',(2.49914305799789,176.002028447915,7.07394587853975));
#1002=CARTESIAN_POINT('Ctrl Pts',(2.35598079328146,175.938139708785,7.12452344672821));
#1003=CARTESIAN_POINT('Ctrl Pts',(2.21093899543762,175.873790551538,7.17087213597972));
#1004=CARTESIAN_POINT('Ctrl Pts',(2.06440202497974,175.809155845315,7.21281294614716));
#1005=CARTESIAN_POINT('Ctrl Pts',(1.91225491695072,175.742046612748,7.25635945154735));
#1006=CARTESIAN_POINT('Ctrl Pts',(1.75849634827299,175.674629757621,7.2951535041046));
#1007=CARTESIAN_POINT('Ctrl Pts',(1.60358071781314,175.607106969111,7.32904872396865));
#1008=CARTESIAN_POINT('Ctrl Pts',(1.4543974295954,175.542082725982,7.36168971919407));
#1009=CARTESIAN_POINT('Ctrl Pts',(1.30414175318146,175.476960494159,7.38978788807506));
#1010=CARTESIAN_POINT('Ctrl Pts',(1.15323346356763,175.411922286781,7.41326371413808));
#1011=CARTESIAN_POINT('Ctrl Pts',(1.0023514247394,175.346895392924,7.43673545653627));
#1012=CARTESIAN_POINT('Ctrl Pts',(0.850817527325577,175.281952719209,7.45558641375475));
#1013=CARTESIAN_POINT('Ctrl Pts',(0.699057151026253,175.217274623013,7.46978884684485));
#1014=CARTESIAN_POINT('Ctrl Pts',(0.547256052215635,175.152579171467,7.4839950909346));
#1015=CARTESIAN_POINT('Ctrl Pts',(0.395228878633319,175.088148656398,7.49355035828583));
#1016=CARTESIAN_POINT('Ctrl Pts',(0.243399260074249,175.024158695687,7.49847872018344));
#1017=CARTESIAN_POINT('Ctrl Pts',(0.225886742935279,175.016777887553,7.49904717331543));
#1018=CARTESIAN_POINT('Ctrl Pts',(0.208376846698734,175.009402933151,7.49955412589778));
#1019=CARTESIAN_POINT('Ctrl Pts',(0.190870214739035,175.002034095791,7.4999996585316));
#1020=CARTESIAN_POINT('',(0.000256710970817156,177.995967593475,7.49999999788466));
#1021=CARTESIAN_POINT('Origin',(-5.20512090547431E-6,178.000081808606,-1851.55088195117));
#1022=CARTESIAN_POINT('',(-1.89809114034451E-16,197.99585953923,7.50000000439337));
#1023=CARTESIAN_POINT('Ctrl Pts',(5.38866871829646E-16,197.99585953923,
7.50000000439337));
#1024=CARTESIAN_POINT('Ctrl Pts',(-1.18775172812192,197.495912211348,7.50000000439337));
#1025=CARTESIAN_POINT('Ctrl Pts',(-2.317383311169,196.995967593475,7.13300320026677));
#1026=CARTESIAN_POINT('Ctrl Pts',(-3.44714003087638,196.495967593475,6.76596574150984));
#1027=CARTESIAN_POINT('Ctrl Pts',(-4.40818170865423,195.995967593475,6.06777834873578));
#1028=CARTESIAN_POINT('Ctrl Pts',(-5.36922338643209,195.495967593475,5.36959095596173));
#1029=CARTESIAN_POINT('Ctrl Pts',(-6.06747656688843,194.995967593475,4.40859707573286));
#1030=CARTESIAN_POINT('Ctrl Pts',(-6.76572974734476,194.495967593475,3.447603195504));
#1031=CARTESIAN_POINT('Ctrl Pts',(-7.13284454416054,193.995967593475,2.31787160445521));
#1032=CARTESIAN_POINT('Ctrl Pts',(-7.49995934097631,193.495967593475,1.18814001340642));
#1033=CARTESIAN_POINT('Ctrl Pts',(-7.5,192.995967593475,0.000256710972401669));
#1034=CARTESIAN_POINT('Ctrl Pts',(-7.50004065902369,192.495967593475,-1.18762659146162));
#1035=CARTESIAN_POINT('Ctrl Pts',(-7.13300320026677,191.995967593475,-2.317383311169));
#1036=CARTESIAN_POINT('Ctrl Pts',(-6.76596574150984,191.495967593475,-3.44714003087638));
#1037=CARTESIAN_POINT('Ctrl Pts',(-6.06777834873578,190.995967593475,-4.40818170865423));
#1038=CARTESIAN_POINT('Ctrl Pts',(-5.36959095596173,190.495967593475,-5.36922338643209));
#1039=CARTESIAN_POINT('Ctrl Pts',(-4.40859707573286,189.995967593475,-6.06747656688843));
#1040=CARTESIAN_POINT('Ctrl Pts',(-3.447603195504,189.495967593475,-6.76572974734476));
#1041=CARTESIAN_POINT('Ctrl Pts',(-2.31787160445521,188.995967593475,-7.13284454416054));
#1042=CARTESIAN_POINT('Ctrl Pts',(-1.18814001340642,188.495967593475,-7.49995934097631));
#1043=CARTESIAN_POINT('Ctrl Pts',(-0.000256710972402128,187.995967593475,
-7.5));
#1044=CARTESIAN_POINT('Ctrl Pts',(1.18762659146162,187.495967593475,-7.50004065902369));
#1045=CARTESIAN_POINT('Ctrl Pts',(2.317383311169,186.995967593475,-7.13300320026677));
#1046=CARTESIAN_POINT('Ctrl Pts',(3.44714003087638,186.495967593475,-6.76596574150984));
#1047=CARTESIAN_POINT('Ctrl Pts',(4.40818170865423,185.995967593475,-6.06777834873578));
#1048=CARTESIAN_POINT('Ctrl Pts',(5.36922338643209,185.495967593475,-5.36959095596173));
#1049=CARTESIAN_POINT('Ctrl Pts',(6.06747656688843,184.995967593475,-4.40859707573286));
#1050=CARTESIAN_POINT('Ctrl Pts',(6.76572974734476,184.495967593475,-3.447603195504));
#1051=CARTESIAN_POINT('Ctrl Pts',(7.13284454416054,183.995967593475,-2.31787160445521));
#1052=CARTESIAN_POINT('Ctrl Pts',(7.49995934097631,183.495967593475,-1.18814001340642));
#1053=CARTESIAN_POINT('Ctrl Pts',(7.5,182.995967593475,-0.000256710972402588));
#1054=CARTESIAN_POINT('Ctrl Pts',(7.50004065902369,182.495967593475,1.18762659146162));
#1055=CARTESIAN_POINT('Ctrl Pts',(7.13300320026677,181.995967593475,2.317383311169));
#1056=CARTESIAN_POINT('Ctrl Pts',(6.76596574150984,181.495967593475,3.44714003087638));
#1057=CARTESIAN_POINT('Ctrl Pts',(6.06777834873579,180.995967593475,4.40818170865423));
#1058=CARTESIAN_POINT('Ctrl Pts',(5.36959095596173,180.495967593475,5.36922338643209));
#1059=CARTESIAN_POINT('Ctrl Pts',(4.40859707573286,179.995967593475,6.06747656688843));
#1060=CARTESIAN_POINT('Ctrl Pts',(3.447603195504,179.495967593475,6.76572974734476));
#1061=CARTESIAN_POINT('Ctrl Pts',(2.31787160445521,178.995967593475,7.13284454416054));
#1062=CARTESIAN_POINT('Ctrl Pts',(1.18814001340643,178.495967593475,7.49995934097631));
#1063=CARTESIAN_POINT('Ctrl Pts',(0.00025671097240121,177.995967593475,
7.5));
#1064=CARTESIAN_POINT('',(-4.06843942354914E-7,214.921557632927,7.50242802810186));
#1065=CARTESIAN_POINT('',(-9.18485099360515E-16,240.,7.5));
#1066=CARTESIAN_POINT('Ctrl Pts',(-4.068439266928E-7,214.921557632927,7.50242802810187));
#1067=CARTESIAN_POINT('Ctrl Pts',(-0.152090385416069,214.857323985265,7.50242801985428));
#1068=CARTESIAN_POINT('Ctrl Pts',(-0.304485788638696,214.792702491972,7.49779895914527));
#1069=CARTESIAN_POINT('Ctrl Pts',(-0.456762644215681,214.72787053402,7.48851081348606));
#1070=CARTESIAN_POINT('Ctrl Pts',(-0.609070650331504,214.663025313709,7.47922076779588));
#1071=CARTESIAN_POINT('Ctrl Pts',(-0.761259533138804,214.597969762788,7.46526968655064));
#1072=CARTESIAN_POINT('Ctrl Pts',(-0.91290272043933,214.532885263597,7.44667945730599));
#1073=CARTESIAN_POINT('Ctrl Pts',(-1.0645049306871,214.467818351553,7.42809425151685));
#1074=CARTESIAN_POINT('Ctrl Pts',(-1.21556121279854,214.402722732839,7.40487246128572));
#1075=CARTESIAN_POINT('Ctrl Pts',(-1.36565093134601,214.3377801784,7.37708776215671));
#1076=CARTESIAN_POINT('Ctrl Pts',(-1.51579830432504,214.272812677376,7.3492923900046));
#1077=CARTESIAN_POINT('Ctrl Pts',(-1.66497786162516,214.207998581557,7.31693074896066));
#1078=CARTESIAN_POINT('Ctrl Pts',(-1.8127818777126,214.143517028959,7.28012693438002));
#1079=CARTESIAN_POINT('Ctrl Pts',(-1.92135204017723,214.096151789321,7.25309251248735));
#1080=CARTESIAN_POINT('Ctrl Pts',(-2.02918025203189,214.04896593395,7.22366229239569));
#1081=CARTESIAN_POINT('Ctrl Pts',(-2.13611185762632,214.002028447915,7.19190186588755));
#1082=CARTESIAN_POINT('Ctrl Pts',(-2.28166131170438,213.938139708658,7.14867131011455));
#1083=CARTESIAN_POINT('Ctrl Pts',(-2.42624566734726,213.87379055128,7.10091475754279));
#1084=CARTESIAN_POINT('Ctrl Pts',(-2.56944875671857,213.809155844927,7.04871331545311));
#1085=CARTESIAN_POINT('Ctrl Pts',(-2.71813540129485,213.74204613624,6.99451296753861));
#1086=CARTESIAN_POINT('Ctrl Pts',(-2.86533230206802,213.674628800623,6.93552054364118));
#1087=CARTESIAN_POINT('Ctrl Pts',(-3.01058579312341,213.607105531561,6.87188471229634));
#1088=CARTESIAN_POINT('Ctrl Pts',(-3.15046347852853,213.542081286575,6.81060403165539));
#1089=CARTESIAN_POINT('Ctrl Pts',(-3.28853853492897,213.476959054234,6.74501779444794));
#1090=CARTESIAN_POINT('Ctrl Pts',(-3.4244246187649,213.411920847683,6.67530840839923));
#1091=CARTESIAN_POINT('Ctrl Pts',(-3.56028706486959,213.346893954694,6.60561114847621));
#1092=CARTESIAN_POINT('Ctrl Pts',(-3.69396084347493,213.281951283189,6.53179244342431));
#1093=CARTESIAN_POINT('Ctrl Pts',(-3.8250855108378,213.217273190526,6.4540798841994));
#1094=CARTESIAN_POINT('Ctrl Pts',(-3.95624536474509,213.152577741871,6.37634647125968));
#1095=CARTESIAN_POINT('Ctrl Pts',(-4.08485433881534,213.088147231023,6.29471745739993));
#1096=CARTESIAN_POINT('Ctrl Pts',(-4.21058385833508,213.02415727582,6.20946132033823));
#1097=CARTESIAN_POINT('Ctrl Pts',(-4.22508868089356,213.016775056042,6.19962572130926));
#1098=CARTESIAN_POINT('Ctrl Pts',(-4.23955521930262,213.009398692253,6.18974188939186));
#1099=CARTESIAN_POINT('Ctrl Pts',(-4.25398300016701,213.002028447915,6.17981026821525));
#1100=CARTESIAN_POINT('Ctrl Pts',(-4.37904978050102,212.938139708658,6.09371831161217));
#1101=CARTESIAN_POINT('Ctrl Pts',(-4.50180008775209,212.87379055128,6.00362010807859));
#1102=CARTESIAN_POINT('Ctrl Pts',(-4.62186318631568,212.809155844927,5.90972139815647));
#1103=CARTESIAN_POINT('Ctrl Pts',(-4.74652375991939,212.74204613624,5.81222710407626));
#1104=CARTESIAN_POINT('Ctrl Pts',(-4.86828667005449,212.674628800623,5.71063563105834));
#1105=CARTESIAN_POINT('Ctrl Pts',(-4.9867663959006,212.607105531561,5.60522856175955));
#1106=CARTESIAN_POINT('Ctrl Pts',(-5.10086120834463,212.542081286575,5.50372258918886));
#1107=CARTESIAN_POINT('Ctrl Pts',(-5.21191112857799,212.476959054234,5.39867883198632));
#1108=CARTESIAN_POINT('Ctrl Pts',(-5.31960508912758,212.411920847683,5.29039015693328));
#1109=CARTESIAN_POINT('Ctrl Pts',(-5.42728031603771,212.346893954693,5.18212031897182));
#1110=CARTESIAN_POINT('Ctrl Pts',(-5.53160039987437,212.281951283189,5.07060708921631));
#1111=CARTESIAN_POINT('Ctrl Pts',(-5.63229286774003,212.217273190525,4.95617830277053));
#1112=CARTESIAN_POINT('Ctrl Pts',(-5.73301235584579,212.152577741871,4.84171881002319));
#1113=CARTESIAN_POINT('Ctrl Pts',(-5.83010200617264,212.088147231022,4.72434264585622));
#1114=CARTESIAN_POINT('Ctrl Pts',(-5.92333228977576,212.02415727582,4.60440668292327));
#1115=CARTESIAN_POINT('Ctrl Pts',(-5.9340878285377,212.016775056041,4.59057023570439));
#1116=CARTESIAN_POINT('Ctrl Pts',(-5.94479205212766,212.009398692253,4.57669974673545));
#1117=CARTESIAN_POINT('Ctrl Pts',(-5.95544464740895,212.002028447915,4.5627957842201));
#1118=CARTESIAN_POINT('Ctrl Pts',(-6.04778634614838,211.938139708658,4.44226970733709));
#1119=CARTESIAN_POINT('Ctrl Pts',(-6.13668694968226,211.87379055128,4.3186492927546));
#1120=CARTESIAN_POINT('Ctrl Pts',(-6.22185744482198,211.809155844927,4.19224477495791));
#1121=CARTESIAN_POINT('Ctrl Pts',(-6.3102893019475,211.74204613624,4.06099995549926));
#1122=CARTESIAN_POINT('Ctrl Pts',(-6.39469921942841,211.674628800622,3.92675391456926));
#1123=CARTESIAN_POINT('Ctrl Pts',(-6.47480755900262,211.607105531561,3.78989358567376));
#1124=CARTESIAN_POINT('Ctrl Pts',(-6.55195110329808,211.542081286575,3.65809843300229));
#1125=CARTESIAN_POINT('Ctrl Pts',(-6.62510554744149,211.476959054234,3.52387957064258));
#1126=CARTESIAN_POINT('Ctrl Pts',(-6.69406554949808,211.411920847683,3.38761165659104));
#1127=CARTESIAN_POINT('Ctrl Pts',(-6.76301355578619,211.346893954693,3.25136744669118));
#1128=CARTESIAN_POINT('Ctrl Pts',(-6.8277683682074,211.281951283189,3.11307538411895));
#1129=CARTESIAN_POINT('Ctrl Pts',(-6.88817215625542,211.217273190525,2.97313145734192));
#1130=CARTESIAN_POINT('Ctrl Pts',(-6.94859215330986,211.152577741871,2.83314997742328));
#1131=CARTESIAN_POINT('Ctrl Pts',(-7.00465866845589,211.088147231022,2.69151625970561));
#1132=CARTESIAN_POINT('Ctrl Pts',(-7.05626368640969,211.02415727582,2.5486406385963));
#1133=CARTESIAN_POINT('Ctrl Pts',(-7.06221711430306,211.016775056041,2.53215775104539));
#1134=CARTESIAN_POINT('Ctrl Pts',(-7.06811121908845,211.009398692253,2.51565834512648));
#1135=CARTESIAN_POINT('Ctrl Pts',(-7.07394587853975,211.002028447915,2.49914305799789));
#1136=CARTESIAN_POINT('Ctrl Pts',(-7.12452344682943,210.938139708658,2.35598079299496));
#1137=CARTESIAN_POINT('Ctrl Pts',(-7.17087213616521,210.87379055128,2.2109389948571));
#1138=CARTESIAN_POINT('Ctrl Pts',(-7.21281294639896,210.809155844927,2.06440202409999));
#1139=CARTESIAN_POINT('Ctrl Pts',(-7.25635976072988,210.74204613624,1.91225383662793));
#1140=CARTESIAN_POINT('Ctrl Pts',(-7.29515405471512,210.674628800622,1.75849416561922));
#1141=CARTESIAN_POINT('Ctrl Pts',(-7.32904944559231,210.607105531561,1.60357741968125));
#1142=CARTESIAN_POINT('Ctrl Pts',(-7.3616903741329,210.542081286575,1.4543941147233));
#1143=CARTESIAN_POINT('Ctrl Pts',(-7.38978847549662,210.476959054234,1.30413842461201));
#1144=CARTESIAN_POINT('Ctrl Pts',(-7.41326423358633,210.411920847683,1.15323012442371));
#1145=CARTESIAN_POINT('Ctrl Pts',(-7.43673590800795,210.346893954693,1.00234807511964));
#1146=CARTESIAN_POINT('Ctrl Pts',(-7.45558679680064,210.281951283189,0.85081417035268));
#1147=CARTESIAN_POINT('Ctrl Pts',(-7.46978916139896,210.217273190525,0.699053789843961));
#1148=CARTESIAN_POINT('Ctrl Pts',(-7.48399533711949,210.152577741871,0.54725268531685));
#1149=CARTESIAN_POINT('Ctrl Pts',(-7.49355053594383,210.088147231022,0.395225509158903));
#1150=CARTESIAN_POINT('Ctrl Pts',(-7.49847882953766,210.02415727582,0.243395891140488));
#1151=CARTESIAN_POINT('Ctrl Pts',(-7.49904738356035,210.016775056041,0.225880023133914));
#1152=CARTESIAN_POINT('Ctrl Pts',(-7.49955441349819,210.009398692253,0.208366777074336));
#1153=CARTESIAN_POINT('Ctrl Pts',(-7.5,210.002028447915,0.190856796705278));
#1154=CARTESIAN_POINT('Ctrl Pts',(-7.50386255306115,209.938139708658,0.0390720635509829));
#1155=CARTESIAN_POINT('Ctrl Pts',(-7.50312239555638,209.87379055128,-0.11319341637498));
#1156=CARTESIAN_POINT('Ctrl Pts',(-7.49772806215971,209.809155844927,-0.265518780411782));
#1157=CARTESIAN_POINT('Ctrl Pts',(-7.49212716810081,209.74204613624,-0.423677011228724));
#1158=CARTESIAN_POINT('Ctrl Pts',(-7.48150838279936,209.674628800622,-0.581899244411169));
#1159=CARTESIAN_POINT('Ctrl Pts',(-7.46587290795738,209.607105531561,-0.739708076930746));
#1160=CARTESIAN_POINT('Ctrl Pts',(-7.4508160992348,209.542081286575,-0.891676432864672));
#1161=CARTESIAN_POINT('Ctrl Pts',(-7.43110741988636,209.476959054234,-1.04326087688651));
#1162=CARTESIAN_POINT('Ctrl Pts',(-7.40680096324212,209.411920847683,-1.19403760734917));
#1163=CARTESIAN_POINT('Ctrl Pts',(-7.38249873476809,209.346893954693,-1.34478810981454));
#1164=CARTESIAN_POINT('Ctrl Pts',(-7.35360044359533,209.281951283189,-1.49473066237887));
#1165=CARTESIAN_POINT('Ctrl Pts',(-7.32021115834334,209.217273190525,-1.64345213319835));
#1166=CARTESIAN_POINT('Ctrl Pts',(-7.28681291327022,209.152577741871,-1.79221351256238));
#1167=CARTESIAN_POINT('Ctrl Pts',(-7.24892146633696,209.088147231022,-1.93975266792269));
#1168=CARTESIAN_POINT('Ctrl Pts',(-7.20669061985644,209.02415727582,-2.08567414197946));
#1169=CARTESIAN_POINT('Ctrl Pts',(-7.20181864597934,209.016775056041,-2.10250841524085));
#1170=CARTESIAN_POINT('Ctrl Pts',(-7.19688896944662,209.009398692253,-2.11932118289467));
#1171=CARTESIAN_POINT('Ctrl Pts',(-7.19190186588755,209.002028447915,-2.13611185762632));
#1172=CARTESIAN_POINT('Ctrl Pts',(-7.14867131011455,208.938139708658,-2.28166131170439));
#1173=CARTESIAN_POINT('Ctrl Pts',(-7.10091475754278,208.87379055128,-2.42624566734729));
#1174=CARTESIAN_POINT('Ctrl Pts',(-7.0487133154531,208.809155844927,-2.56944875671861));
#1175=CARTESIAN_POINT('Ctrl Pts',(-6.99451296753859,208.74204613624,-2.71813540129489));
#1176=CARTESIAN_POINT('Ctrl Pts',(-6.93552054364117,208.674628800623,-2.86533230206806));
#1177=CARTESIAN_POINT('Ctrl Pts',(-6.87188471229632,208.607105531561,-3.01058579312345));
#1178=CARTESIAN_POINT('Ctrl Pts',(-6.8106040316553,208.542081286575,-3.15046347852873));
#1179=CARTESIAN_POINT('Ctrl Pts',(-6.74501779444778,208.476959054234,-3.28853853492931));
#1180=CARTESIAN_POINT('Ctrl Pts',(-6.67530840839898,208.411920847683,-3.42442461876539));
#1181=CARTESIAN_POINT('Ctrl Pts',(-6.60561114847592,208.346893954693,-3.56028706487013));
#1182=CARTESIAN_POINT('Ctrl Pts',(-6.53179244342397,208.281951283189,-3.69396084347553));
#1183=CARTESIAN_POINT('Ctrl Pts',(-6.45407988419901,208.217273190525,-3.82508551083845));
#1184=CARTESIAN_POINT('Ctrl Pts',(-6.37634647125933,208.152577741871,-3.95624536474565));
#1185=CARTESIAN_POINT('Ctrl Pts',(-6.29471745739962,208.088147231022,-4.08485433881581));
#1186=CARTESIAN_POINT('Ctrl Pts',(-6.20946132033797,208.02415727582,-4.21058385833547));
#1187=CARTESIAN_POINT('Ctrl Pts',(-6.19962572130909,208.016775056041,-4.22508868089382));
#1188=CARTESIAN_POINT('Ctrl Pts',(-6.18974188939178,208.009398692253,-4.23955521930275));
#1189=CARTESIAN_POINT('Ctrl Pts',(-6.17981026821526,208.002028447915,-4.253983000167));
#1190=CARTESIAN_POINT('Ctrl Pts',(-6.09371831161218,207.938139708658,-4.379049780501));
#1191=CARTESIAN_POINT('Ctrl Pts',(-6.00362010807862,207.87379055128,-4.50180008775205));
#1192=CARTESIAN_POINT('Ctrl Pts',(-5.90972139815651,207.809155844927,-4.62186318631563));
#1193=CARTESIAN_POINT('Ctrl Pts',(-5.81222710407629,207.74204613624,-4.74652375991935));
#1194=CARTESIAN_POINT('Ctrl Pts',(-5.71063563105837,207.674628800623,-4.86828667005446));
#1195=CARTESIAN_POINT('Ctrl Pts',(-5.60522856175958,207.607105531561,-4.98676639590057));
#1196=CARTESIAN_POINT('Ctrl Pts',(-5.50372258918887,207.542081286575,-5.10086120834461));
#1197=CARTESIAN_POINT('Ctrl Pts',(-5.39867883198632,207.476959054234,-5.21191112857799));
#1198=CARTESIAN_POINT('Ctrl Pts',(-5.29039015693326,207.411920847683,-5.3196050891276));
#1199=CARTESIAN_POINT('Ctrl Pts',(-5.18212031897177,207.346893954693,-5.42728031603775));
#1200=CARTESIAN_POINT('Ctrl Pts',(-5.07060708921622,207.281951283189,-5.53160039987444));
#1201=CARTESIAN_POINT('Ctrl Pts',(-4.95617830277041,207.217273190525,-5.63229286774013));
#1202=CARTESIAN_POINT('Ctrl Pts',(-4.8417188100227,207.152577741871,-5.73301235584621));
#1203=CARTESIAN_POINT('Ctrl Pts',(-4.72434264585535,207.088147231022,-5.83010200617336));
#1204=CARTESIAN_POINT('Ctrl Pts',(-4.60440668292199,207.024157275819,-5.92333228977675));
#1205=CARTESIAN_POINT('Ctrl Pts',(-4.59057023570353,207.016775056041,-5.93408782853836));
#1206=CARTESIAN_POINT('Ctrl Pts',(-4.57669974673502,207.009398692253,-5.94479205212799));
#1207=CARTESIAN_POINT('Ctrl Pts',(-4.56279578422009,207.002028447915,-5.95544464740895));
#1208=CARTESIAN_POINT('Ctrl Pts',(-4.44226970733713,206.938139708658,-6.04778634614835));
#1209=CARTESIAN_POINT('Ctrl Pts',(-4.31864929275468,206.87379055128,-6.1366869496822));
#1210=CARTESIAN_POINT('Ctrl Pts',(-4.19224477495804,206.809155844927,-6.22185744482189));
#1211=CARTESIAN_POINT('Ctrl Pts',(-4.06099995549939,206.74204613624,-6.31028930194741));
#1212=CARTESIAN_POINT('Ctrl Pts',(-3.92675391456938,206.674628800622,-6.39469921942834));
#1213=CARTESIAN_POINT('Ctrl Pts',(-3.78989358567387,206.607105531561,-6.47480755900256));
#1214=CARTESIAN_POINT('Ctrl Pts',(-3.65809843300235,206.542081286575,-6.55195110329805));
#1215=CARTESIAN_POINT('Ctrl Pts',(-3.52387957064261,206.476959054234,-6.62510554744148));
#1216=CARTESIAN_POINT('Ctrl Pts',(-3.38761165659103,206.411920847683,-6.69406554949809));
#1217=CARTESIAN_POINT('Ctrl Pts',(-3.25136744669109,206.346893954693,-6.76301355578624));
#1218=CARTESIAN_POINT('Ctrl Pts',(-3.11307538411878,206.281951283189,-6.82776836820748));
#1219=CARTESIAN_POINT('Ctrl Pts',(-2.97313145734166,206.217273190525,-6.88817215625554));
#1220=CARTESIAN_POINT('Ctrl Pts',(-2.8331499774231,206.152577741871,-6.94859215330993));
#1221=CARTESIAN_POINT('Ctrl Pts',(-2.69151625970553,206.088147231022,-7.00465866845592));
#1222=CARTESIAN_POINT('Ctrl Pts',(-2.54864063859631,206.02415727582,-7.05626368640968));
#1223=CARTESIAN_POINT('Ctrl Pts',(-2.53215775104539,206.016775056041,-7.06221711430306));
#1224=CARTESIAN_POINT('Ctrl Pts',(-2.51565834512647,206.009398692253,-7.06811121908845));
#1225=CARTESIAN_POINT('Ctrl Pts',(-2.49914305799788,206.002028447915,-7.07394587853976));
#1226=CARTESIAN_POINT('Ctrl Pts',(-2.35598079299498,205.938139708658,-7.12452344682942));
#1227=CARTESIAN_POINT('Ctrl Pts',(-2.21093899485714,205.87379055128,-7.1708721361652));
#1228=CARTESIAN_POINT('Ctrl Pts',(-2.06440202410006,205.809155844927,-7.21281294639894));
#1229=CARTESIAN_POINT('Ctrl Pts',(-1.91225383662799,205.74204613624,-7.25635976072986));
#1230=CARTESIAN_POINT('Ctrl Pts',(-1.75849416561927,205.674628800623,-7.29515405471511));
#1231=CARTESIAN_POINT('Ctrl Pts',(-1.60357741968129,205.607105531561,-7.32904944559231));
#1232=CARTESIAN_POINT('Ctrl Pts',(-1.45439411472333,205.542081286575,-7.36169037413289));
#1233=CARTESIAN_POINT('Ctrl Pts',(-1.30413842461202,205.476959054234,-7.38978847549662));
#1234=CARTESIAN_POINT('Ctrl Pts',(-1.15323012442371,205.411920847683,-7.41326423358633));
#1235=CARTESIAN_POINT('Ctrl Pts',(-1.00234807511963,205.346893954693,-7.43673590800795));
#1236=CARTESIAN_POINT('Ctrl Pts',(-0.850814170352673,205.281951283189,-7.45558679680064));
#1237=CARTESIAN_POINT('Ctrl Pts',(-0.699053789843954,205.217273190525,-7.46978916139896));
#1238=CARTESIAN_POINT('Ctrl Pts',(-0.547252685316885,205.152577741871,-7.48399533711949));
#1239=CARTESIAN_POINT('Ctrl Pts',(-0.39522550915898,205.088147231022,-7.49355053594382));
#1240=CARTESIAN_POINT('Ctrl Pts',(-0.243395891140606,205.02415727582,-7.49847882953766));
#1241=CARTESIAN_POINT('Ctrl Pts',(-0.225880023133996,205.016775056041,-7.49904738356035));
#1242=CARTESIAN_POINT('Ctrl Pts',(-0.208366777074381,205.009398692253,-7.49955441349818));
#1243=CARTESIAN_POINT('Ctrl Pts',(-0.190856796705286,205.002028447915,-7.5));
#1244=CARTESIAN_POINT('Ctrl Pts',(-0.0390720635510205,204.938139708658,
-7.50386255306115));
#1245=CARTESIAN_POINT('Ctrl Pts',(0.113193416374905,204.87379055128,-7.50312239555638));
#1246=CARTESIAN_POINT('Ctrl Pts',(0.265518780411678,204.809155844927,-7.49772806215972));
#1247=CARTESIAN_POINT('Ctrl Pts',(0.42367701122863,204.74204613624,-7.49212716810082));
#1248=CARTESIAN_POINT('Ctrl Pts',(0.581899244411101,204.674628800623,-7.48150838279936));
#1249=CARTESIAN_POINT('Ctrl Pts',(0.739708076930687,204.607105531561,-7.46587290795739));
#1250=CARTESIAN_POINT('Ctrl Pts',(0.891676432865158,204.542081286575,-7.45081609923475));
#1251=CARTESIAN_POINT('Ctrl Pts',(1.04326087688753,204.476959054234,-7.43110741988623));
#1252=CARTESIAN_POINT('Ctrl Pts',(1.19403760735073,204.411920847682,-7.40680096324187));
#1253=CARTESIAN_POINT('Ctrl Pts',(1.34478810981601,204.346893954693,-7.38249873476782));
#1254=CARTESIAN_POINT('Ctrl Pts',(1.49473066238024,204.281951283188,-7.35360044359504));
#1255=CARTESIAN_POINT('Ctrl Pts',(1.64345213319964,204.217273190525,-7.32021115834305));
#1256=CARTESIAN_POINT('Ctrl Pts',(1.79221351256366,204.15257774187,-7.28681291326991));
#1257=CARTESIAN_POINT('Ctrl Pts',(1.93975266792397,204.088147231022,-7.24892146633662));
#1258=CARTESIAN_POINT('Ctrl Pts',(2.08567414198074,204.024157275819,-7.20669061985607));
#1259=CARTESIAN_POINT('Ctrl Pts',(2.1025084152417,204.016775056041,-7.20181864597909));
#1260=CARTESIAN_POINT('Ctrl Pts',(2.1193211828951,204.009398692253,-7.19688896944649));
#1261=CARTESIAN_POINT('Ctrl Pts',(2.13611185762632,204.002028447915,-7.19190186588755));
#1262=CARTESIAN_POINT('Ctrl Pts',(2.28166131170441,203.938139708658,-7.14867131011454));
#1263=CARTESIAN_POINT('Ctrl Pts',(2.42624566734732,203.87379055128,-7.10091475754277));
#1264=CARTESIAN_POINT('Ctrl Pts',(2.56944875671865,203.809155844927,-7.04871331545308));
#1265=CARTESIAN_POINT('Ctrl Pts',(2.71813540129493,203.74204613624,-6.99451296753857));
#1266=CARTESIAN_POINT('Ctrl Pts',(2.86533230206809,203.674628800623,-6.93552054364115));
#1267=CARTESIAN_POINT('Ctrl Pts',(3.01058579312348,203.607105531561,-6.87188471229631));
#1268=CARTESIAN_POINT('Ctrl Pts',(3.15046347852877,203.542081286575,-6.81060403165528));
#1269=CARTESIAN_POINT('Ctrl Pts',(3.28853853492937,203.476959054234,-6.74501779444775));
#1270=CARTESIAN_POINT('Ctrl Pts',(3.42442461876546,203.411920847683,-6.67530840839894));
#1271=CARTESIAN_POINT('Ctrl Pts',(3.56028706487072,203.346893954693,-6.60561114847562));
#1272=CARTESIAN_POINT('Ctrl Pts',(3.69396084347661,203.281951283188,-6.53179244342338));
#1273=CARTESIAN_POINT('Ctrl Pts',(3.82508551084001,203.217273190525,-6.45407988419809));
#1274=CARTESIAN_POINT('Ctrl Pts',(3.95624536474729,203.15257774187,-6.37634647125832));
#1275=CARTESIAN_POINT('Ctrl Pts',(4.08485433881753,203.088147231021,-6.29471745739851));
#1276=CARTESIAN_POINT('Ctrl Pts',(4.21058385833727,203.024157275819,-6.20946132033675));
#1277=CARTESIAN_POINT('Ctrl Pts',(4.22508868089501,203.016775056041,-6.19962572130827));
#1278=CARTESIAN_POINT('Ctrl Pts',(4.23955521930334,203.009398692253,-6.18974188939137));
#1279=CARTESIAN_POINT('Ctrl Pts',(4.25398300016701,203.002028447915,-6.17981026821526));
#1280=CARTESIAN_POINT('Ctrl Pts',(4.37904978050104,202.938139708658,-6.09371831161216));
#1281=CARTESIAN_POINT('Ctrl Pts',(4.50180008775212,202.87379055128,-6.00362010807857));
#1282=CARTESIAN_POINT('Ctrl Pts',(4.62186318631574,202.809155844927,-5.90972139815643));
#1283=CARTESIAN_POINT('Ctrl Pts',(4.74652375991944,202.74204613624,-5.81222710407621));
#1284=CARTESIAN_POINT('Ctrl Pts',(4.86828667005455,202.674628800622,-5.71063563105829));
#1285=CARTESIAN_POINT('Ctrl Pts',(4.98676639590066,202.607105531561,-5.60522856175951));
#1286=CARTESIAN_POINT('Ctrl Pts',(5.10086120834481,202.542081286575,-5.50372258918869));
#1287=CARTESIAN_POINT('Ctrl Pts',(5.21191112857829,202.476959054234,-5.39867883198603));
#1288=CARTESIAN_POINT('Ctrl Pts',(5.319605089128,202.411920847683,-5.29039015693286));
#1289=CARTESIAN_POINT('Ctrl Pts',(5.42728031603811,202.346893954693,-5.1821203189714));
#1290=CARTESIAN_POINT('Ctrl Pts',(5.53160039987475,202.281951283188,-5.07060708921589));
#1291=CARTESIAN_POINT('Ctrl Pts',(5.6322928677404,202.217273190525,-4.95617830277011));
#1292=CARTESIAN_POINT('Ctrl Pts',(5.73301235584613,202.152577741871,-4.84171881002279));
#1293=CARTESIAN_POINT('Ctrl Pts',(5.83010200617296,202.088147231022,-4.72434264585582));
#1294=CARTESIAN_POINT('Ctrl Pts',(5.92333228977606,202.024157275819,-4.60440668292288));
#1295=CARTESIAN_POINT('Ctrl Pts',(5.93408782853791,202.016775056041,-4.59057023570412));
#1296=CARTESIAN_POINT('Ctrl Pts',(5.94479205212776,202.009398692253,-4.57669974673532));
#1297=CARTESIAN_POINT('Ctrl Pts',(5.95544464740895,202.002028447915,-4.56279578422009));
#1298=CARTESIAN_POINT('Ctrl Pts',(6.04778634614835,201.938139708658,-4.44226970733712));
#1299=CARTESIAN_POINT('Ctrl Pts',(6.13668694968221,201.87379055128,-4.31864929275467));
#1300=CARTESIAN_POINT('Ctrl Pts',(6.22185744482191,201.809155844927,-4.19224477495801));
#1301=CARTESIAN_POINT('Ctrl Pts',(6.31028930194743,201.74204613624,-4.06099995549936));
#1302=CARTESIAN_POINT('Ctrl Pts',(6.39469921942835,201.674628800622,-3.92675391456936));
#1303=CARTESIAN_POINT('Ctrl Pts',(6.47480755900257,201.607105531561,-3.78989358567385));
#1304=CARTESIAN_POINT('Ctrl Pts',(6.55195110329815,201.542081286575,-3.65809843300218));
#1305=CARTESIAN_POINT('Ctrl Pts',(6.62510554744167,201.476959054234,-3.52387957064226));
#1306=CARTESIAN_POINT('Ctrl Pts',(6.69406554949835,201.411920847682,-3.38761165659051));
#1307=CARTESIAN_POINT('Ctrl Pts',(6.76301355578675,201.346893954693,-3.25136744669006));
#1308=CARTESIAN_POINT('Ctrl Pts',(6.8277683682082,201.281951283188,-3.11307538411724));
#1309=CARTESIAN_POINT('Ctrl Pts',(6.88817215625643,201.217273190524,-2.97313145733959));
#1310=CARTESIAN_POINT('Ctrl Pts',(6.94859215331078,201.15257774187,-2.83314997742101));
#1311=CARTESIAN_POINT('Ctrl Pts',(7.00465866845674,201.088147231021,-2.69151625970341));
#1312=CARTESIAN_POINT('Ctrl Pts',(7.05626368641046,201.024157275819,-2.54864063859417));
#1313=CARTESIAN_POINT('Ctrl Pts',(7.06221711430357,201.016775056041,-2.53215775104397));
#1314=CARTESIAN_POINT('Ctrl Pts',(7.0681112190887,201.009398692253,-2.51565834512576));
#1315=CARTESIAN_POINT('Ctrl Pts',(7.07394587853975,201.002028447915,-2.49914305799789));
#1316=CARTESIAN_POINT('Ctrl Pts',(7.12452344682944,200.938139708658,-2.35598079299493));
#1317=CARTESIAN_POINT('Ctrl Pts',(7.17087213616524,200.87379055128,-2.21093899485702));
#1318=CARTESIAN_POINT('Ctrl Pts',(7.21281294639899,200.809155844927,-2.06440202409988));
#1319=CARTESIAN_POINT('Ctrl Pts',(7.25635976072991,200.74204613624,-1.91225383662782));
#1320=CARTESIAN_POINT('Ctrl Pts',(7.29515405471514,200.674628800622,-1.75849416561912));
#1321=CARTESIAN_POINT('Ctrl Pts',(7.32904944559233,200.607105531561,-1.60357741968116));
#1322=CARTESIAN_POINT('Ctrl Pts',(7.36169037413292,200.542081286575,-1.45439411472321));
#1323=CARTESIAN_POINT('Ctrl Pts',(7.38978847549664,200.476959054234,-1.30413842461191));
#1324=CARTESIAN_POINT('Ctrl Pts',(7.41326423358634,200.411920847683,-1.15323012442361));
#1325=CARTESIAN_POINT('Ctrl Pts',(7.43673590800806,200.346893954693,-1.00234807511895));
#1326=CARTESIAN_POINT('Ctrl Pts',(7.4555867968008,200.281951283188,-0.850814170351404));
#1327=CARTESIAN_POINT('Ctrl Pts',(7.46978916139914,200.217273190525,-0.699053789842093));
#1328=CARTESIAN_POINT('Ctrl Pts',(7.48399533711963,200.15257774187,-0.547252685315009));
#1329=CARTESIAN_POINT('Ctrl Pts',(7.49355053594392,200.088147231021,-0.395225509157083));
#1330=CARTESIAN_POINT('Ctrl Pts',(7.49847882953772,200.024157275819,-0.243395891138698));
#1331=CARTESIAN_POINT('Ctrl Pts',(7.49904738356038,200.016775056041,-0.225880023132722));
#1332=CARTESIAN_POINT('Ctrl Pts',(7.4995544134982,200.009398692253,-0.208366777073748));
#1333=CARTESIAN_POINT('Ctrl Pts',(7.5,200.002028447915,-0.190856796705287));
#1334=CARTESIAN_POINT('Ctrl Pts',(7.50386255306115,199.938139708658,-0.0390720635509912));
#1335=CARTESIAN_POINT('Ctrl Pts',(7.50312239555638,199.87379055128,0.113193416374972));
#1336=CARTESIAN_POINT('Ctrl Pts',(7.49772806215971,199.809155844927,0.265518780411775));
#1337=CARTESIAN_POINT('Ctrl Pts',(7.49212716810081,199.74204613624,0.423677011228717));
#1338=CARTESIAN_POINT('Ctrl Pts',(7.48150838279936,199.674628800623,0.581899244411163));
#1339=CARTESIAN_POINT('Ctrl Pts',(7.46587290795738,199.607105531561,0.73970807693074));
#1340=CARTESIAN_POINT('Ctrl Pts',(7.4508160992348,199.542081286575,0.891676432864664));
#1341=CARTESIAN_POINT('Ctrl Pts',(7.43110741988637,199.476959054234,1.04326087688649));
#1342=CARTESIAN_POINT('Ctrl Pts',(7.40680096324213,199.411920847683,1.19403760734915));
#1343=CARTESIAN_POINT('Ctrl Pts',(7.38249873476819,199.346893954694,1.34478810981391));
#1344=CARTESIAN_POINT('Ctrl Pts',(7.35360044359557,199.281951283189,1.49473066237762));
#1345=CARTESIAN_POINT('Ctrl Pts',(7.32021115834376,199.217273190526,1.64345213319651));
#1346=CARTESIAN_POINT('Ctrl Pts',(7.28681291327069,199.152577741872,1.79221351256049));
#1347=CARTESIAN_POINT('Ctrl Pts',(7.24892146633748,199.088147231023,1.93975266792075));
#1348=CARTESIAN_POINT('Ctrl Pts',(7.20669061985702,199.02415727582,2.08567414197748));
#1349=CARTESIAN_POINT('Ctrl Pts',(7.20181864597973,199.016775056042,2.10250841523952));
#1350=CARTESIAN_POINT('Ctrl Pts',(7.19688896944681,199.009398692254,2.11932118289401));
#1351=CARTESIAN_POINT('Ctrl Pts',(7.19190186588755,199.002028447915,2.13611185762632));
#1352=CARTESIAN_POINT('Ctrl Pts',(7.14867131011454,198.938139708658,2.28166131170442));
#1353=CARTESIAN_POINT('Ctrl Pts',(7.10091475754276,198.87379055128,2.42624566734735));
#1354=CARTESIAN_POINT('Ctrl Pts',(7.04871331545307,198.809155844927,2.56944875671869));
#1355=CARTESIAN_POINT('Ctrl Pts',(6.99451296753856,198.74204613624,2.71813540129497));
#1356=CARTESIAN_POINT('Ctrl Pts',(6.93552054364114,198.674628800622,2.86533230206812));
#1357=CARTESIAN_POINT('Ctrl Pts',(6.8718847122963,198.607105531561,3.0105857931235));
#1358=CARTESIAN_POINT('Ctrl Pts',(6.81060403165536,198.542081286575,3.1504634785286));
#1359=CARTESIAN_POINT('Ctrl Pts',(6.74501779444792,198.476959054234,3.288538534929));
#1360=CARTESIAN_POINT('Ctrl Pts',(6.67530840839923,198.411920847683,3.42442461876491));
#1361=CARTESIAN_POINT('Ctrl Pts',(6.60561114847646,198.346893954694,3.56028706486911));
#1362=CARTESIAN_POINT('Ctrl Pts',(6.53179244342483,198.281951283189,3.69396084347398));
#1363=CARTESIAN_POINT('Ctrl Pts',(6.45407988420023,198.217273190526,3.8250855108364));
#1364=CARTESIAN_POINT('Ctrl Pts',(6.37634647126055,198.152577741872,3.9562453647437));
#1365=CARTESIAN_POINT('Ctrl Pts',(6.29471745740083,198.088147231023,4.08485433881396));
#1366=CARTESIAN_POINT('Ctrl Pts',(6.20946132033916,198.024157275821,4.21058385833372));
#1367=CARTESIAN_POINT('Ctrl Pts',(6.19962572130989,198.016775056042,4.22508868089265));
#1368=CARTESIAN_POINT('Ctrl Pts',(6.18974188939218,198.009398692254,4.23955521930217));
#1369=CARTESIAN_POINT('Ctrl Pts',(6.17981026821526,198.002028447915,4.25398300016701));
#1370=CARTESIAN_POINT('Ctrl Pts',(6.09371831161217,197.938139708658,4.37904978050101));
#1371=CARTESIAN_POINT('Ctrl Pts',(6.0036201080786,197.87379055128,4.50180008775207));
#1372=CARTESIAN_POINT('Ctrl Pts',(5.90972139815648,197.809155844927,4.62186318631566));
#1373=CARTESIAN_POINT('Ctrl Pts',(5.81222710407627,197.74204613624,4.74652375991938));
#1374=CARTESIAN_POINT('Ctrl Pts',(5.71063563105834,197.674628800623,4.86828667005449));
#1375=CARTESIAN_POINT('Ctrl Pts',(5.60522856175956,197.607105531561,4.9867663959006));
#1376=CARTESIAN_POINT('Ctrl Pts',(5.50372258918911,197.542081286575,5.10086120834435));
#1377=CARTESIAN_POINT('Ctrl Pts',(5.39867883198685,197.476959054235,5.21191112857743));
#1378=CARTESIAN_POINT('Ctrl Pts',(5.29039015693409,197.411920847683,5.31960508912677));
#1379=CARTESIAN_POINT('Ctrl Pts',(5.18212031897387,197.346893954695,5.4272803160357));
#1380=CARTESIAN_POINT('Ctrl Pts',(5.07060708921967,197.281951283191,5.53160039987124));
#1381=CARTESIAN_POINT('Ctrl Pts',(4.95617830277527,197.217273190528,5.63229286773586));
#1382=CARTESIAN_POINT('Ctrl Pts',(4.84171881002731,197.152577741873,5.73301235584234));
#1383=CARTESIAN_POINT('Ctrl Pts',(4.72434264585968,197.088147231024,5.83010200616986));
#1384=CARTESIAN_POINT('Ctrl Pts',(4.60440668292603,197.024157275821,5.92333228977361));
#1385=CARTESIAN_POINT('Ctrl Pts',(4.59057023570623,197.016775056042,5.93408782853628));
#1386=CARTESIAN_POINT('Ctrl Pts',(4.57669974673637,197.009398692254,5.94479205212695));
#1387=CARTESIAN_POINT('Ctrl Pts',(4.56279578422009,197.002028447915,5.95544464740895));
#1388=CARTESIAN_POINT('Ctrl Pts',(4.44226970733712,196.938139708658,6.04778634614835));
#1389=CARTESIAN_POINT('Ctrl Pts',(4.31864929275467,196.87379055128,6.13668694968221));
#1390=CARTESIAN_POINT('Ctrl Pts',(4.19224477495802,196.809155844927,6.22185744482191));
#1391=CARTESIAN_POINT('Ctrl Pts',(4.06099995549936,196.74204613624,6.31028930194743));
#1392=CARTESIAN_POINT('Ctrl Pts',(3.92675391456935,196.674628800622,6.39469921942835));
#1393=CARTESIAN_POINT('Ctrl Pts',(3.78989358567384,196.607105531561,6.47480755900257));
#1394=CARTESIAN_POINT('Ctrl Pts',(3.6580984330025,196.542081286575,6.55195110329796));
#1395=CARTESIAN_POINT('Ctrl Pts',(3.52387957064293,196.476959054234,6.62510554744131));
#1396=CARTESIAN_POINT('Ctrl Pts',(3.38761165659153,196.411920847683,6.69406554949784));
#1397=CARTESIAN_POINT('Ctrl Pts',(3.25136744669109,196.346893954693,6.76301355578625));
#1398=CARTESIAN_POINT('Ctrl Pts',(3.11307538411827,196.281951283188,6.82776836820773));
#1399=CARTESIAN_POINT('Ctrl Pts',(2.97313145734063,196.217273190525,6.88817215625598));
#1400=CARTESIAN_POINT('Ctrl Pts',(2.83314997742163,196.15257774187,6.94859215331054));
#1401=CARTESIAN_POINT('Ctrl Pts',(2.69151625970362,196.088147231021,7.00465866845667));
#1402=CARTESIAN_POINT('Ctrl Pts',(2.54864063859395,196.024157275819,7.05626368641054));
#1403=CARTESIAN_POINT('Ctrl Pts',(2.53215775104383,196.016775056041,7.06221711430362));
#1404=CARTESIAN_POINT('Ctrl Pts',(2.51565834512569,196.009398692253,7.06811121908872));
#1405=CARTESIAN_POINT('Ctrl Pts',(2.49914305799789,196.002028447915,7.07394587853975));
#1406=CARTESIAN_POINT('Ctrl Pts',(2.35598079299495,195.938139708658,7.12452344682943));
#1407=CARTESIAN_POINT('Ctrl Pts',(2.21093899485708,195.87379055128,7.17087213616522));
#1408=CARTESIAN_POINT('Ctrl Pts',(2.06440202409996,195.809155844927,7.21281294639897));
#1409=CARTESIAN_POINT('Ctrl Pts',(1.9122538366279,195.74204613624,7.25635976072989));
#1410=CARTESIAN_POINT('Ctrl Pts',(1.75849416561919,195.674628800623,7.29515405471513));
#1411=CARTESIAN_POINT('Ctrl Pts',(1.60357741968122,195.607105531561,7.32904944559232));
#1412=CARTESIAN_POINT('Ctrl Pts',(1.4543941147231,195.542081286575,7.36169037413294));
#1413=CARTESIAN_POINT('Ctrl Pts',(1.30413842461163,195.476959054234,7.38978847549669));
#1414=CARTESIAN_POINT('Ctrl Pts',(1.15323012442317,195.411920847683,7.41326423358641));
#1415=CARTESIAN_POINT('Ctrl Pts',(1.00234807511844,195.346893954693,7.43673590800813));
#1416=CARTESIAN_POINT('Ctrl Pts',(0.850814170350841,195.281951283188,7.45558679680086));
#1417=CARTESIAN_POINT('Ctrl Pts',(0.69905378984147,195.217273190524,7.46978916139919));
#1418=CARTESIAN_POINT('Ctrl Pts',(0.547252685314392,195.15257774187,7.48399533711967));
#1419=CARTESIAN_POINT('Ctrl Pts',(0.395225509156497,195.088147231021,7.49355053594395));
#1420=CARTESIAN_POINT('Ctrl Pts',(0.243395891138119,195.024157275819,7.49847882953774));
#1421=CARTESIAN_POINT('Ctrl Pts',(0.225880023132343,195.016775056041,7.4990473835604));
#1422=CARTESIAN_POINT('Ctrl Pts',(0.208366777073546,195.009398692253,7.49955441349821));
#1423=CARTESIAN_POINT('Ctrl Pts',(0.190856796705285,195.002028447915,7.5));
#1424=CARTESIAN_POINT('Ctrl Pts',(0.127311648028404,194.975281229334,7.50161706980302));
#1425=CARTESIAN_POINT('Ctrl Pts',(0.0636823578853578,194.948453397593,7.50242803155527));
#1426=CARTESIAN_POINT('Ctrl Pts',(-4.06843965232862E-7,194.921557632927,
7.50242802810186));
#1427=CARTESIAN_POINT('Origin',(0.,400.,3.5527136788005E-14));
#1428=CARTESIAN_POINT('Origin',(0.,240.,0.));
#1429=CARTESIAN_POINT('Ctrl Pts',(5.38002895896315E-16,217.99585953923,
7.50000000439337));
#1430=CARTESIAN_POINT('Ctrl Pts',(-1.18775172812189,217.495912211348,7.50000000439337));
#1431=CARTESIAN_POINT('Ctrl Pts',(-2.317383311169,216.995967593475,7.13300320026677));
#1432=CARTESIAN_POINT('Ctrl Pts',(-3.44714003087638,216.495967593475,6.76596574150984));
#1433=CARTESIAN_POINT('Ctrl Pts',(-4.40818170865423,215.995967593475,6.06777834873578));
#1434=CARTESIAN_POINT('Ctrl Pts',(-5.36922338643209,215.495967593475,5.36959095596173));
#1435=CARTESIAN_POINT('Ctrl Pts',(-6.06747656688843,214.995967593475,4.40859707573286));
#1436=CARTESIAN_POINT('Ctrl Pts',(-6.76572974734476,214.495967593475,3.447603195504));
#1437=CARTESIAN_POINT('Ctrl Pts',(-7.13284454416054,213.995967593475,2.31787160445521));
#1438=CARTESIAN_POINT('Ctrl Pts',(-7.49995934097631,213.495967593475,1.18814001340642));
#1439=CARTESIAN_POINT('Ctrl Pts',(-7.5,212.995967593475,0.000256710972401669));
#1440=CARTESIAN_POINT('Ctrl Pts',(-7.50004065902369,212.495967593475,-1.18762659146162));
#1441=CARTESIAN_POINT('Ctrl Pts',(-7.13300320026677,211.995967593475,-2.317383311169));
#1442=CARTESIAN_POINT('Ctrl Pts',(-6.76596574150984,211.495967593475,-3.44714003087638));
#1443=CARTESIAN_POINT('Ctrl Pts',(-6.06777834873578,210.995967593475,-4.40818170865423));
#1444=CARTESIAN_POINT('Ctrl Pts',(-5.36959095596173,210.495967593475,-5.36922338643209));
#1445=CARTESIAN_POINT('Ctrl Pts',(-4.40859707573286,209.995967593475,-6.06747656688843));
#1446=CARTESIAN_POINT('Ctrl Pts',(-3.447603195504,209.495967593475,-6.76572974734476));
#1447=CARTESIAN_POINT('Ctrl Pts',(-2.31787160445521,208.995967593475,-7.13284454416054));
#1448=CARTESIAN_POINT('Ctrl Pts',(-1.18814001340642,208.495967593475,-7.49995934097631));
#1449=CARTESIAN_POINT('Ctrl Pts',(-0.000256710972402128,207.995967593475,
-7.5));
#1450=CARTESIAN_POINT('Ctrl Pts',(1.18762659146162,207.495967593475,-7.50004065902369));
#1451=CARTESIAN_POINT('Ctrl Pts',(2.317383311169,206.995967593475,-7.13300320026677));
#1452=CARTESIAN_POINT('Ctrl Pts',(3.44714003087638,206.495967593475,-6.76596574150984));
#1453=CARTESIAN_POINT('Ctrl Pts',(4.40818170865423,205.995967593475,-6.06777834873578));
#1454=CARTESIAN_POINT('Ctrl Pts',(5.36922338643209,205.495967593475,-5.36959095596173));
#1455=CARTESIAN_POINT('Ctrl Pts',(6.06747656688843,204.995967593475,-4.40859707573286));
#1456=CARTESIAN_POINT('Ctrl Pts',(6.76572974734476,204.495967593475,-3.447603195504));
#1457=CARTESIAN_POINT('Ctrl Pts',(7.13284454416054,203.995967593475,-2.31787160445521));
#1458=CARTESIAN_POINT('Ctrl Pts',(7.49995934097631,203.495967593475,-1.18814001340642));
#1459=CARTESIAN_POINT('Ctrl Pts',(7.5,202.995967593475,-0.000256710972402588));
#1460=CARTESIAN_POINT('Ctrl Pts',(7.50004065902369,202.495967593475,1.18762659146162));
#1461=CARTESIAN_POINT('Ctrl Pts',(7.13300320026677,201.995967593475,2.317383311169));
#1462=CARTESIAN_POINT('Ctrl Pts',(6.76596574150984,201.495967593475,3.44714003087638));
#1463=CARTESIAN_POINT('Ctrl Pts',(6.06777834873579,200.995967593475,4.40818170865423));
#1464=CARTESIAN_POINT('Ctrl Pts',(5.36959095596173,200.495967593475,5.36922338643209));
#1465=CARTESIAN_POINT('Ctrl Pts',(4.40859707573286,199.995967593475,6.06747656688843));
#1466=CARTESIAN_POINT('Ctrl Pts',(3.447603195504,199.495967593475,6.76572974734476));
#1467=CARTESIAN_POINT('Ctrl Pts',(2.31787160445521,198.995967593475,7.13284454416054));
#1468=CARTESIAN_POINT('Ctrl Pts',(1.18814001340643,198.495967593475,7.49995934097631));
#1469=CARTESIAN_POINT('Ctrl Pts',(0.00025671097240121,197.995967593475,
7.5));
#1470=CARTESIAN_POINT('Ctrl Pts',(0.000128355486237033,197.995913566499,
7.50000000439337));
#1471=CARTESIAN_POINT('Ctrl Pts',(5.38866871829646E-16,197.99585953923,
7.50000000439337));
#1472=CARTESIAN_POINT('Ctrl Pts',(-4.06843934450864E-7,234.921557632927,
7.50242802810186));
#1473=CARTESIAN_POINT('Ctrl Pts',(-0.152090385416014,234.857323985265,7.50242801985428));
#1474=CARTESIAN_POINT('Ctrl Pts',(-0.304485788638578,234.792702491972,7.49779895914527));
#1475=CARTESIAN_POINT('Ctrl Pts',(-0.456762644215501,234.72787053402,7.48851081348607));
#1476=CARTESIAN_POINT('Ctrl Pts',(-0.609070650331329,234.663025313709,7.4792207677959));
#1477=CARTESIAN_POINT('Ctrl Pts',(-0.761259533138642,234.597969762788,7.46526968655066));
#1478=CARTESIAN_POINT('Ctrl Pts',(-0.912902720439174,234.532885263597,7.44667945730601));
#1479=CARTESIAN_POINT('Ctrl Pts',(-1.06450493068721,234.467818351553,7.42809425151684));
#1480=CARTESIAN_POINT('Ctrl Pts',(-1.2155612127989,234.402722732839,7.40487246128567));
#1481=CARTESIAN_POINT('Ctrl Pts',(-1.36565093134662,234.3377801784,7.3770877621566));
#1482=CARTESIAN_POINT('Ctrl Pts',(-1.51579830432564,234.272812677376,7.34929239000448));
#1483=CARTESIAN_POINT('Ctrl Pts',(-1.66497786162574,234.207998581557,7.31693074896052));
#1484=CARTESIAN_POINT('Ctrl Pts',(-1.81278187771317,234.143517028959,7.28012693437987));
#1485=CARTESIAN_POINT('Ctrl Pts',(-1.92135204017761,234.096151789321,7.25309251248725));
#1486=CARTESIAN_POINT('Ctrl Pts',(-2.02918025203209,234.04896593395,7.22366229239563));
#1487=CARTESIAN_POINT('Ctrl Pts',(-2.13611185762633,234.002028447915,7.19190186588755));
#1488=CARTESIAN_POINT('Ctrl Pts',(-2.28166131170441,233.938139708658,7.14867131011454));
#1489=CARTESIAN_POINT('Ctrl Pts',(-2.42624566734732,233.87379055128,7.10091475754277));
#1490=CARTESIAN_POINT('Ctrl Pts',(-2.56944875671866,233.809155844927,7.04871331545308));
#1491=CARTESIAN_POINT('Ctrl Pts',(-2.71813540129493,233.74204613624,6.99451296753857));
#1492=CARTESIAN_POINT('Ctrl Pts',(-2.8653323020681,233.674628800622,6.93552054364115));
#1493=CARTESIAN_POINT('Ctrl Pts',(-3.01058579312348,233.607105531561,6.8718847122963));
#1494=CARTESIAN_POINT('Ctrl Pts',(-3.15046347852879,233.542081286575,6.81060403165527));
#1495=CARTESIAN_POINT('Ctrl Pts',(-3.28853853492939,233.476959054234,6.74501779444774));
#1496=CARTESIAN_POINT('Ctrl Pts',(-3.42442461876549,233.411920847683,6.67530840839893));
#1497=CARTESIAN_POINT('Ctrl Pts',(-3.56028706487034,233.346893954693,6.60561114847581));
#1498=CARTESIAN_POINT('Ctrl Pts',(-3.69396084347583,233.281951283188,6.5317924434238));
#1499=CARTESIAN_POINT('Ctrl Pts',(-3.82508551083885,233.217273190525,6.45407988419878));
#1500=CARTESIAN_POINT('Ctrl Pts',(-3.95624536474616,233.152577741871,6.37634647125902));
#1501=CARTESIAN_POINT('Ctrl Pts',(-4.08485433881642,233.088147231022,6.29471745739923));
#1502=CARTESIAN_POINT('Ctrl Pts',(-4.21058385833618,233.024157275819,6.20946132033749));
#1503=CARTESIAN_POINT('Ctrl Pts',(-4.22508868089429,233.016775056041,6.19962572130877));
#1504=CARTESIAN_POINT('Ctrl Pts',(-4.23955521930298,233.009398692253,6.18974188939162));
#1505=CARTESIAN_POINT('Ctrl Pts',(-4.25398300016701,233.002028447915,6.17981026821526));
#1506=CARTESIAN_POINT('Ctrl Pts',(-4.3790497805011,232.938139708658,6.09371831161211));
#1507=CARTESIAN_POINT('Ctrl Pts',(-4.50180008775226,232.87379055128,6.00362010807847));
#1508=CARTESIAN_POINT('Ctrl Pts',(-4.62186318631593,232.809155844927,5.90972139815627));
#1509=CARTESIAN_POINT('Ctrl Pts',(-4.74652375991963,232.74204613624,5.81222710407607));
#1510=CARTESIAN_POINT('Ctrl Pts',(-4.86828667005471,232.674628800622,5.71063563105815));
#1511=CARTESIAN_POINT('Ctrl Pts',(-4.9867663959008,232.607105531561,5.60522856175938));
#1512=CARTESIAN_POINT('Ctrl Pts',(-5.10086120834483,232.542081286575,5.50372258918868));
#1513=CARTESIAN_POINT('Ctrl Pts',(-5.21191112857818,232.476959054234,5.39867883198613));
#1514=CARTESIAN_POINT('Ctrl Pts',(-5.31960508912778,232.411920847683,5.29039015693308));
#1515=CARTESIAN_POINT('Ctrl Pts',(-5.4272803160379,232.346893954693,5.18212031897162));
#1516=CARTESIAN_POINT('Ctrl Pts',(-5.53160039987455,232.281951283189,5.07060708921611));
#1517=CARTESIAN_POINT('Ctrl Pts',(-5.63229286774021,232.217273190525,4.95617830277033));
#1518=CARTESIAN_POINT('Ctrl Pts',(-5.7330123558459,232.152577741871,4.84171881002306));
#1519=CARTESIAN_POINT('Ctrl Pts',(-5.83010200617269,232.088147231022,4.72434264585615));
#1520=CARTESIAN_POINT('Ctrl Pts',(-5.92333228977576,232.02415727582,4.60440668292327));
#1521=CARTESIAN_POINT('Ctrl Pts',(-5.9340878285377,232.016775056041,4.59057023570438));
#1522=CARTESIAN_POINT('Ctrl Pts',(-5.94479205212766,232.009398692253,4.57669974673544));
#1523=CARTESIAN_POINT('Ctrl Pts',(-5.95544464740896,232.002028447915,4.56279578422008));
#1524=CARTESIAN_POINT('Ctrl Pts',(-6.04778634614836,231.938139708658,4.44226970733711));
#1525=CARTESIAN_POINT('Ctrl Pts',(-6.13668694968222,231.87379055128,4.31864929275465));
#1526=CARTESIAN_POINT('Ctrl Pts',(-6.22185744482192,231.809155844927,4.192244774958));
#1527=CARTESIAN_POINT('Ctrl Pts',(-6.31028930194744,231.74204613624,4.06099995549935));
#1528=CARTESIAN_POINT('Ctrl Pts',(-6.39469921942836,231.674628800622,3.92675391456934));
#1529=CARTESIAN_POINT('Ctrl Pts',(-6.47480755900258,231.607105531561,3.78989358567383));
#1530=CARTESIAN_POINT('Ctrl Pts',(-6.55195110329806,231.542081286575,3.65809843300233));
#1531=CARTESIAN_POINT('Ctrl Pts',(-6.62510554744149,231.476959054234,3.52387957064259));
#1532=CARTESIAN_POINT('Ctrl Pts',(-6.6940655494981,231.411920847683,3.38761165659102));
#1533=CARTESIAN_POINT('Ctrl Pts',(-6.76301355578627,231.346893954693,3.25136744669103));
#1534=CARTESIAN_POINT('Ctrl Pts',(-6.82776836820753,231.281951283188,3.11307538411867));
#1535=CARTESIAN_POINT('Ctrl Pts',(-6.8881721562556,231.217273190525,2.97313145734151));
#1536=CARTESIAN_POINT('Ctrl Pts',(-6.94859215330999,231.152577741871,2.83314997742295));
#1537=CARTESIAN_POINT('Ctrl Pts',(-7.00465866845598,231.088147231022,2.69151625970537));
#1538=CARTESIAN_POINT('Ctrl Pts',(-7.05626368640974,231.024157275819,2.54864063859615));
#1539=CARTESIAN_POINT('Ctrl Pts',(-7.06221711430309,231.016775056041,2.53215775104529));
#1540=CARTESIAN_POINT('Ctrl Pts',(-7.06811121908846,231.009398692253,2.51565834512643));
#1541=CARTESIAN_POINT('Ctrl Pts',(-7.07394587853975,231.002028447915,2.49914305799789));
#1542=CARTESIAN_POINT('Ctrl Pts',(-7.12452344682943,230.938139708658,2.35598079299495));
#1543=CARTESIAN_POINT('Ctrl Pts',(-7.17087213616522,230.87379055128,2.21093899485707));
#1544=CARTESIAN_POINT('Ctrl Pts',(-7.21281294639897,230.809155844927,2.06440202409995));
#1545=CARTESIAN_POINT('Ctrl Pts',(-7.25635976072989,230.74204613624,1.91225383662789));
#1546=CARTESIAN_POINT('Ctrl Pts',(-7.29515405471513,230.674628800623,1.75849416561917));
#1547=CARTESIAN_POINT('Ctrl Pts',(-7.32904944559233,230.607105531561,1.6035774196812));
#1548=CARTESIAN_POINT('Ctrl Pts',(-7.36169037413292,230.542081286575,1.45439411472321));
#1549=CARTESIAN_POINT('Ctrl Pts',(-7.38978847549665,230.476959054234,1.30413842461186));
#1550=CARTESIAN_POINT('Ctrl Pts',(-7.41326423358636,230.411920847683,1.15323012442351));
#1551=CARTESIAN_POINT('Ctrl Pts',(-7.43673590800799,230.346893954693,1.00234807511941));
#1552=CARTESIAN_POINT('Ctrl Pts',(-7.45558679680067,230.281951283188,0.850814170352427));
#1553=CARTESIAN_POINT('Ctrl Pts',(-7.46978916139899,230.217273190525,0.699053789843682));
#1554=CARTESIAN_POINT('Ctrl Pts',(-7.48399533711951,230.152577741871,0.547252685316623));
#1555=CARTESIAN_POINT('Ctrl Pts',(-7.49355053594384,230.088147231022,0.395225509158728));
#1556=CARTESIAN_POINT('Ctrl Pts',(-7.49847882953767,230.02415727582,0.243395891140365));
#1557=CARTESIAN_POINT('Ctrl Pts',(-7.49904738356035,230.016775056041,0.225880023133833));
#1558=CARTESIAN_POINT('Ctrl Pts',(-7.49955441349819,230.009398692253,0.208366777074296));
#1559=CARTESIAN_POINT('Ctrl Pts',(-7.5,230.002028447915,0.19085679670528));
#1560=CARTESIAN_POINT('Ctrl Pts',(-7.50386255306115,229.938139708658,0.0390720635509798));
#1561=CARTESIAN_POINT('Ctrl Pts',(-7.50312239555638,229.87379055128,-0.113193416374988));
#1562=CARTESIAN_POINT('Ctrl Pts',(-7.49772806215971,229.809155844927,-0.265518780411795));
#1563=CARTESIAN_POINT('Ctrl Pts',(-7.49212716810081,229.74204613624,-0.423677011228737));
#1564=CARTESIAN_POINT('Ctrl Pts',(-7.48150838279935,229.674628800622,-0.581899244411182));
#1565=CARTESIAN_POINT('Ctrl Pts',(-7.46587290795738,229.607105531561,-0.739708076930759));
#1566=CARTESIAN_POINT('Ctrl Pts',(-7.4508160992348,229.542081286575,-0.891676432864674));
#1567=CARTESIAN_POINT('Ctrl Pts',(-7.43110741988637,229.476959054234,-1.0432608768865));
#1568=CARTESIAN_POINT('Ctrl Pts',(-7.40680096324213,229.411920847683,-1.19403760734915));
#1569=CARTESIAN_POINT('Ctrl Pts',(-7.38249873476809,229.346893954693,-1.34478810981454));
#1570=CARTESIAN_POINT('Ctrl Pts',(-7.35360044359533,229.281951283189,-1.49473066237887));
#1571=CARTESIAN_POINT('Ctrl Pts',(-7.32021115834334,229.217273190525,-1.64345213319836));
#1572=CARTESIAN_POINT('Ctrl Pts',(-7.28681291327022,229.152577741871,-1.79221351256241));
#1573=CARTESIAN_POINT('Ctrl Pts',(-7.24892146633694,229.088147231022,-1.93975266792275));
#1574=CARTESIAN_POINT('Ctrl Pts',(-7.20669061985642,229.02415727582,-2.08567414197955));
#1575=CARTESIAN_POINT('Ctrl Pts',(-7.20181864597933,229.016775056041,-2.1025084152409));
#1576=CARTESIAN_POINT('Ctrl Pts',(-7.19688896944661,229.009398692253,-2.1193211828947));
#1577=CARTESIAN_POINT('Ctrl Pts',(-7.19190186588755,229.002028447915,-2.13611185762632));
#1578=CARTESIAN_POINT('Ctrl Pts',(-7.14867131011454,228.938139708658,-2.28166131170441));
#1579=CARTESIAN_POINT('Ctrl Pts',(-7.10091475754277,228.87379055128,-2.42624566734733));
#1580=CARTESIAN_POINT('Ctrl Pts',(-7.04871331545307,228.809155844927,-2.56944875671868));
#1581=CARTESIAN_POINT('Ctrl Pts',(-6.99451296753857,228.74204613624,-2.71813540129495));
#1582=CARTESIAN_POINT('Ctrl Pts',(-6.93552054364114,228.674628800622,-2.86533230206812));
#1583=CARTESIAN_POINT('Ctrl Pts',(-6.8718847122963,228.607105531561,-3.0105857931235));
#1584=CARTESIAN_POINT('Ctrl Pts',(-6.81060403165529,228.542081286575,-3.15046347852874));
#1585=CARTESIAN_POINT('Ctrl Pts',(-6.74501779444778,228.476959054234,-3.2885385349293));
#1586=CARTESIAN_POINT('Ctrl Pts',(-6.675308408399,228.411920847683,-3.42442461876534));
#1587=CARTESIAN_POINT('Ctrl Pts',(-6.60561114847594,228.346893954693,-3.5602870648701));
#1588=CARTESIAN_POINT('Ctrl Pts',(-6.53179244342398,228.281951283189,-3.69396084347551));
#1589=CARTESIAN_POINT('Ctrl Pts',(-6.45407988419902,228.217273190525,-3.82508551083845));
#1590=CARTESIAN_POINT('Ctrl Pts',(-6.37634647125928,228.152577741871,-3.95624536474574));
#1591=CARTESIAN_POINT('Ctrl Pts',(-6.29471745739952,228.088147231022,-4.08485433881598));
#1592=CARTESIAN_POINT('Ctrl Pts',(-6.2094613203378,228.02415727582,-4.21058385833573));
#1593=CARTESIAN_POINT('Ctrl Pts',(-6.19962572130897,228.016775056041,-4.22508868089399));
#1594=CARTESIAN_POINT('Ctrl Pts',(-6.18974188939172,228.009398692253,-4.23955521930283));
#1595=CARTESIAN_POINT('Ctrl Pts',(-6.17981026821526,228.002028447915,-4.25398300016701));
#1596=CARTESIAN_POINT('Ctrl Pts',(-6.09371831161215,227.938139708658,-4.37904978050104));
#1597=CARTESIAN_POINT('Ctrl Pts',(-6.00362010807856,227.87379055128,-4.50180008775213));
#1598=CARTESIAN_POINT('Ctrl Pts',(-5.90972139815641,227.809155844927,-4.62186318631575));
#1599=CARTESIAN_POINT('Ctrl Pts',(-5.8122271040762,227.74204613624,-4.74652375991946));
#1600=CARTESIAN_POINT('Ctrl Pts',(-5.71063563105828,227.674628800622,-4.86828667005456));
#1601=CARTESIAN_POINT('Ctrl Pts',(-5.6052285617595,227.607105531561,-4.98676639590066));
#1602=CARTESIAN_POINT('Ctrl Pts',(-5.50372258918886,227.542081286575,-5.10086120834462));
#1603=CARTESIAN_POINT('Ctrl Pts',(-5.39867883198638,227.476959054234,-5.21191112857791));
#1604=CARTESIAN_POINT('Ctrl Pts',(-5.29039015693341,227.411920847683,-5.31960508912745));
#1605=CARTESIAN_POINT('Ctrl Pts',(-5.18212031897197,227.346893954694,-5.42728031603756));
#1606=CARTESIAN_POINT('Ctrl Pts',(-5.07060708921648,227.281951283189,-5.5316003998742));
#1607=CARTESIAN_POINT('Ctrl Pts',(-4.95617830277073,227.217273190526,-5.63229286773986));
#1608=CARTESIAN_POINT('Ctrl Pts',(-4.84171881002346,227.152577741871,-5.73301235584555));
#1609=CARTESIAN_POINT('Ctrl Pts',(-4.72434264585657,227.088147231022,-5.83010200617235));
#1610=CARTESIAN_POINT('Ctrl Pts',(-4.60440668292369,227.02415727582,-5.92333228977543));
#1611=CARTESIAN_POINT('Ctrl Pts',(-4.59057023570467,227.016775056041,-5.93408782853748));
#1612=CARTESIAN_POINT('Ctrl Pts',(-4.57669974673559,227.009398692253,-5.94479205212755));
#1613=CARTESIAN_POINT('Ctrl Pts',(-4.56279578422009,227.002028447915,-5.95544464740895));
#1614=CARTESIAN_POINT('Ctrl Pts',(-4.44226970733717,226.938139708658,-6.04778634614832));
#1615=CARTESIAN_POINT('Ctrl Pts',(-4.31864929275475,226.87379055128,-6.13668694968215));
#1616=CARTESIAN_POINT('Ctrl Pts',(-4.19224477495815,226.809155844927,-6.22185744482182));
#1617=CARTESIAN_POINT('Ctrl Pts',(-4.06099995549949,226.74204613624,-6.31028930194735));
#1618=CARTESIAN_POINT('Ctrl Pts',(-3.92675391456947,226.674628800623,-6.39469921942828));
#1619=CARTESIAN_POINT('Ctrl Pts',(-3.78989358567395,226.607105531561,-6.47480755900251));
#1620=CARTESIAN_POINT('Ctrl Pts',(-3.65809843300246,226.542081286575,-6.55195110329799));
#1621=CARTESIAN_POINT('Ctrl Pts',(-3.52387957064274,226.476959054234,-6.62510554744141));
#1622=CARTESIAN_POINT('Ctrl Pts',(-3.38761165659118,226.411920847683,-6.69406554949802));
#1623=CARTESIAN_POINT('Ctrl Pts',(-3.25136744669125,226.346893954693,-6.76301355578616));
#1624=CARTESIAN_POINT('Ctrl Pts',(-3.11307538411895,226.281951283189,-6.8277683682074));
#1625=CARTESIAN_POINT('Ctrl Pts',(-2.97313145734185,226.217273190525,-6.88817215625545));
#1626=CARTESIAN_POINT('Ctrl Pts',(-2.83314997742316,226.152577741871,-6.94859215330991));
#1627=CARTESIAN_POINT('Ctrl Pts',(-2.69151625970544,226.088147231022,-7.00465866845596));
#1628=CARTESIAN_POINT('Ctrl Pts',(-2.54864063859608,226.024157275819,-7.05626368640977));
#1629=CARTESIAN_POINT('Ctrl Pts',(-2.53215775104524,226.016775056041,-7.06221711430311));
#1630=CARTESIAN_POINT('Ctrl Pts',(-2.5156583451264,226.009398692253,-7.06811121908847));
#1631=CARTESIAN_POINT('Ctrl Pts',(-2.49914305799788,226.002028447915,-7.07394587853975));
#1632=CARTESIAN_POINT('Ctrl Pts',(-2.35598079299495,225.938139708658,-7.12452344682943));
#1633=CARTESIAN_POINT('Ctrl Pts',(-2.21093899485708,225.87379055128,-7.17087213616522));
#1634=CARTESIAN_POINT('Ctrl Pts',(-2.06440202409996,225.809155844927,-7.21281294639897));
#1635=CARTESIAN_POINT('Ctrl Pts',(-1.9122538366279,225.74204613624,-7.25635976072989));
#1636=CARTESIAN_POINT('Ctrl Pts',(-1.75849416561919,225.674628800623,-7.29515405471513));
#1637=CARTESIAN_POINT('Ctrl Pts',(-1.60357741968122,225.607105531561,-7.32904944559232));
#1638=CARTESIAN_POINT('Ctrl Pts',(-1.45439411472326,225.542081286575,-7.36169037413291));
#1639=CARTESIAN_POINT('Ctrl Pts',(-1.30413842461196,225.476959054234,-7.38978847549663));
#1640=CARTESIAN_POINT('Ctrl Pts',(-1.15323012442366,225.411920847683,-7.41326423358633));
#1641=CARTESIAN_POINT('Ctrl Pts',(-1.00234807511957,225.346893954693,-7.43673590800797));
#1642=CARTESIAN_POINT('Ctrl Pts',(-0.850814170352588,225.281951283189,-7.45558679680065));
#1643=CARTESIAN_POINT('Ctrl Pts',(-0.699053789843849,225.217273190525,-7.46978916139897));
#1644=CARTESIAN_POINT('Ctrl Pts',(-0.547252685316753,225.152577741871,-7.4839953371195));
#1645=CARTESIAN_POINT('Ctrl Pts',(-0.395225509158822,225.088147231022,-7.49355053594383));
#1646=CARTESIAN_POINT('Ctrl Pts',(-0.243395891140422,225.02415727582,-7.49847882953767));
#1647=CARTESIAN_POINT('Ctrl Pts',(-0.225880023133874,225.016775056041,-7.49904738356035));
#1648=CARTESIAN_POINT('Ctrl Pts',(-0.208366777074322,225.009398692253,-7.49955441349819));
#1649=CARTESIAN_POINT('Ctrl Pts',(-0.19085679670529,225.002028447915,-7.5));
#1650=CARTESIAN_POINT('Ctrl Pts',(-0.0390720635510056,224.938139708658,
-7.50386255306115));
#1651=CARTESIAN_POINT('Ctrl Pts',(0.113193416374946,224.87379055128,-7.50312239555638));
#1652=CARTESIAN_POINT('Ctrl Pts',(0.265518780411738,224.809155844927,-7.49772806215971));
#1653=CARTESIAN_POINT('Ctrl Pts',(0.423677011228685,224.74204613624,-7.49212716810082));
#1654=CARTESIAN_POINT('Ctrl Pts',(0.581899244411136,224.674628800623,-7.48150838279936));
#1655=CARTESIAN_POINT('Ctrl Pts',(0.739708076930718,224.607105531561,-7.46587290795738));
#1656=CARTESIAN_POINT('Ctrl Pts',(0.891676432864649,224.542081286575,-7.4508160992348));
#1657=CARTESIAN_POINT('Ctrl Pts',(1.04326087688649,224.476959054234,-7.43110741988637));
#1658=CARTESIAN_POINT('Ctrl Pts',(1.19403760734915,224.411920847683,-7.40680096324213));
#1659=CARTESIAN_POINT('Ctrl Pts',(1.34478810981431,224.346893954693,-7.38249873476812));
#1660=CARTESIAN_POINT('Ctrl Pts',(1.49473066237841,224.281951283189,-7.35360044359541));
#1661=CARTESIAN_POINT('Ctrl Pts',(1.64345213319768,224.217273190526,-7.32021115834349));
#1662=CARTESIAN_POINT('Ctrl Pts',(1.79221351256174,224.152577741871,-7.28681291327038));
#1663=CARTESIAN_POINT('Ctrl Pts',(1.93975266792208,224.088147231022,-7.24892146633712));
#1664=CARTESIAN_POINT('Ctrl Pts',(2.08567414197888,224.02415727582,-7.20669061985661));
#1665=CARTESIAN_POINT('Ctrl Pts',(2.10250841524046,224.016775056041,-7.20181864597946));
#1666=CARTESIAN_POINT('Ctrl Pts',(2.11932118289448,224.009398692253,-7.19688896944667));
#1667=CARTESIAN_POINT('Ctrl Pts',(2.13611185762633,224.002028447915,-7.19190186588755));
#1668=CARTESIAN_POINT('Ctrl Pts',(2.28166131170461,223.938139708658,-7.14867131011448));
#1669=CARTESIAN_POINT('Ctrl Pts',(2.42624566734772,223.87379055128,-7.10091475754264));
#1670=CARTESIAN_POINT('Ctrl Pts',(2.56944875671925,223.809155844927,-7.04871331545287));
#1671=CARTESIAN_POINT('Ctrl Pts',(2.71813540129546,223.74204613624,-6.99451296753837));
#1672=CARTESIAN_POINT('Ctrl Pts',(2.86533230206858,223.674628800622,-6.93552054364095));
#1673=CARTESIAN_POINT('Ctrl Pts',(3.01058579312391,223.60710553156,-6.87188471229612));
#1674=CARTESIAN_POINT('Ctrl Pts',(3.1504634785292,223.542081286575,-6.81060403165508));
#1675=CARTESIAN_POINT('Ctrl Pts',(3.2885385349298,223.476959054234,-6.74501779444754));
#1676=CARTESIAN_POINT('Ctrl Pts',(3.42442461876589,223.411920847683,-6.67530840839872));
#1677=CARTESIAN_POINT('Ctrl Pts',(3.56028706487057,223.346893954693,-6.60561114847569));
#1678=CARTESIAN_POINT('Ctrl Pts',(3.69396084347589,223.281951283188,-6.53179244342376));
#1679=CARTESIAN_POINT('Ctrl Pts',(3.82508551083875,223.217273190525,-6.45407988419884));
#1680=CARTESIAN_POINT('Ctrl Pts',(3.95624536474612,223.152577741871,-6.37634647125905));
#1681=CARTESIAN_POINT('Ctrl Pts',(4.08485433881643,223.088147231022,-6.29471745739922));
#1682=CARTESIAN_POINT('Ctrl Pts',(4.21058385833625,223.024157275819,-6.20946132033745));
#1683=CARTESIAN_POINT('Ctrl Pts',(4.22508868089433,223.016775056041,-6.19962572130874));
#1684=CARTESIAN_POINT('Ctrl Pts',(4.239555219303,223.009398692253,-6.1897418893916));
#1685=CARTESIAN_POINT('Ctrl Pts',(4.253983000167,223.002028447915,-6.17981026821526));
#1686=CARTESIAN_POINT('Ctrl Pts',(4.379049780501,222.938139708658,-6.09371831161218));
#1687=CARTESIAN_POINT('Ctrl Pts',(4.50180008775205,222.87379055128,-6.00362010807862));
#1688=CARTESIAN_POINT('Ctrl Pts',(4.62186318631563,222.809155844927,-5.90972139815651));
#1689=CARTESIAN_POINT('Ctrl Pts',(4.74652375991935,222.74204613624,-5.81222710407629));
#1690=CARTESIAN_POINT('Ctrl Pts',(4.86828667005446,222.674628800623,-5.71063563105837));
#1691=CARTESIAN_POINT('Ctrl Pts',(4.98676639590057,222.607105531561,-5.60522856175958));
#1692=CARTESIAN_POINT('Ctrl Pts',(5.10086120834461,222.542081286575,-5.50372258918887));
#1693=CARTESIAN_POINT('Ctrl Pts',(5.21191112857799,222.476959054234,-5.39867883198631));
#1694=CARTESIAN_POINT('Ctrl Pts',(5.3196050891276,222.411920847683,-5.29039015693326));
#1695=CARTESIAN_POINT('Ctrl Pts',(5.42728031603795,222.346893954693,-5.18212031897158));
#1696=CARTESIAN_POINT('Ctrl Pts',(5.53160039987481,222.281951283188,-5.07060708921584));
#1697=CARTESIAN_POINT('Ctrl Pts',(5.63229286774066,222.217273190525,-4.95617830276981));
#1698=CARTESIAN_POINT('Ctrl Pts',(5.73301235584641,222.152577741871,-4.84171881002245));
#1699=CARTESIAN_POINT('Ctrl Pts',(5.83010200617326,222.088147231022,-4.72434264585545));
#1700=CARTESIAN_POINT('Ctrl Pts',(5.92333228977638,222.024157275819,-4.60440668292247));
#1701=CARTESIAN_POINT('Ctrl Pts',(5.93408782853811,222.016775056041,-4.59057023570385));
#1702=CARTESIAN_POINT('Ctrl Pts',(5.94479205212787,222.009398692253,-4.57669974673517));
#1703=CARTESIAN_POINT('Ctrl Pts',(5.95544464740896,222.002028447915,-4.56279578422009));
#1704=CARTESIAN_POINT('Ctrl Pts',(6.04778634614835,221.938139708658,-4.44226970733712));
#1705=CARTESIAN_POINT('Ctrl Pts',(6.13668694968221,221.87379055128,-4.31864929275467));
#1706=CARTESIAN_POINT('Ctrl Pts',(6.2218574448219,221.809155844927,-4.19224477495803));
#1707=CARTESIAN_POINT('Ctrl Pts',(6.31028930194743,221.74204613624,-4.06099995549937));
#1708=CARTESIAN_POINT('Ctrl Pts',(6.39469921942835,221.674628800622,-3.92675391456936));
#1709=CARTESIAN_POINT('Ctrl Pts',(6.47480755900257,221.607105531561,-3.78989358567385));
#1710=CARTESIAN_POINT('Ctrl Pts',(6.55195110329805,221.542081286575,-3.65809843300234));
#1711=CARTESIAN_POINT('Ctrl Pts',(6.62510554744149,221.476959054234,-3.5238795706426));
#1712=CARTESIAN_POINT('Ctrl Pts',(6.6940655494981,221.411920847683,-3.38761165659102));
#1713=CARTESIAN_POINT('Ctrl Pts',(6.76301355578647,221.346893954693,-3.25136744669064));
#1714=CARTESIAN_POINT('Ctrl Pts',(6.8277683682079,221.281951283188,-3.11307538411788));
#1715=CARTESIAN_POINT('Ctrl Pts',(6.88817215625612,221.217273190525,-2.9731314573403));
#1716=CARTESIAN_POINT('Ctrl Pts',(6.94859215331057,221.15257774187,-2.83314997742154));
#1717=CARTESIAN_POINT('Ctrl Pts',(7.00465866845661,221.088147231021,-2.69151625970376));
#1718=CARTESIAN_POINT('Ctrl Pts',(7.0562636864104,221.024157275819,-2.54864063859434));
#1719=CARTESIAN_POINT('Ctrl Pts',(7.06221711430353,221.016775056041,-2.53215775104408));
#1720=CARTESIAN_POINT('Ctrl Pts',(7.06811121908868,221.009398692253,-2.51565834512583));
#1721=CARTESIAN_POINT('Ctrl Pts',(7.07394587853975,221.002028447915,-2.4991430579979));
#1722=CARTESIAN_POINT('Ctrl Pts',(7.12452344682937,220.938139708658,-2.35598079299513));
#1723=CARTESIAN_POINT('Ctrl Pts',(7.17087213616511,220.87379055128,-2.21093899485743));
#1724=CARTESIAN_POINT('Ctrl Pts',(7.21281294639882,220.809155844927,-2.06440202410049));
#1725=CARTESIAN_POINT('Ctrl Pts',(7.25635976072976,220.74204613624,-1.91225383662838));
#1726=CARTESIAN_POINT('Ctrl Pts',(7.29515405471502,220.674628800623,-1.75849416561964));
#1727=CARTESIAN_POINT('Ctrl Pts',(7.32904944559223,220.607105531561,-1.60357741968163));
#1728=CARTESIAN_POINT('Ctrl Pts',(7.36169037413284,220.542081286575,-1.4543941147236));
#1729=CARTESIAN_POINT('Ctrl Pts',(7.38978847549659,220.476959054234,-1.30413842461222));
#1730=CARTESIAN_POINT('Ctrl Pts',(7.41326423358631,220.411920847683,-1.15323012442383));
#1731=CARTESIAN_POINT('Ctrl Pts',(7.43673590800786,220.346893954694,-1.00234807512029));
#1732=CARTESIAN_POINT('Ctrl Pts',(7.4555867968005,220.281951283189,-0.850814170353856));
#1733=CARTESIAN_POINT('Ctrl Pts',(7.4697891613988,220.217273190526,-0.69905378984567));
#1734=CARTESIAN_POINT('Ctrl Pts',(7.48399533711939,220.152577741872,-0.547252685318368));
#1735=CARTESIAN_POINT('Ctrl Pts',(7.49355053594376,220.088147231023,-0.395225509160228));
#1736=CARTESIAN_POINT('Ctrl Pts',(7.49847882953763,220.02415727582,-0.243395891141619));
#1737=CARTESIAN_POINT('Ctrl Pts',(7.49904738356033,220.016775056042,-0.22588002313467));
#1738=CARTESIAN_POINT('Ctrl Pts',(7.49955441349818,220.009398692253,-0.20836677707472));
#1739=CARTESIAN_POINT('Ctrl Pts',(7.5,220.002028447915,-0.190856796705287));
#1740=CARTESIAN_POINT('Ctrl Pts',(7.50386255306115,219.938139708658,-0.0390720635509813));
#1741=CARTESIAN_POINT('Ctrl Pts',(7.50312239555638,219.87379055128,0.113193416374992));
#1742=CARTESIAN_POINT('Ctrl Pts',(7.49772806215971,219.809155844927,0.265518780411804));
#1743=CARTESIAN_POINT('Ctrl Pts',(7.49212716810081,219.74204613624,0.423677011228746));
#1744=CARTESIAN_POINT('Ctrl Pts',(7.48150838279935,219.674628800622,0.581899244411192));
#1745=CARTESIAN_POINT('Ctrl Pts',(7.46587290795738,219.607105531561,0.739708076930769));
#1746=CARTESIAN_POINT('Ctrl Pts',(7.45081609923482,219.542081286575,0.891676432864501));
#1747=CARTESIAN_POINT('Ctrl Pts',(7.43110741988641,219.476959054234,1.04326087688616));
#1748=CARTESIAN_POINT('Ctrl Pts',(7.40680096324221,219.411920847683,1.19403760734863));
#1749=CARTESIAN_POINT('Ctrl Pts',(7.38249873476801,219.346893954693,1.34478810981507));
#1750=CARTESIAN_POINT('Ctrl Pts',(7.35360044359503,219.281951283188,1.49473066238045));
#1751=CARTESIAN_POINT('Ctrl Pts',(7.32021115834276,219.217273190524,1.64345213320097));
#1752=CARTESIAN_POINT('Ctrl Pts',(7.28681291326939,219.152577741869,1.79221351256585));
#1753=CARTESIAN_POINT('Ctrl Pts',(7.24892146633583,219.08814723102,1.93975266792699));
#1754=CARTESIAN_POINT('Ctrl Pts',(7.20669061985496,219.024157275817,2.08567414198458));
#1755=CARTESIAN_POINT('Ctrl Pts',(7.20181864597834,219.01677505604,2.10250841524425));
#1756=CARTESIAN_POINT('Ctrl Pts',(7.19688896944612,219.009398692252,2.11932118289636));
#1757=CARTESIAN_POINT('Ctrl Pts',(7.19190186588756,219.002028447915,2.13611185762631));
#1758=CARTESIAN_POINT('Ctrl Pts',(7.14867131011454,218.938139708658,2.28166131170442));
#1759=CARTESIAN_POINT('Ctrl Pts',(7.10091475754276,218.87379055128,2.42624566734735));
#1760=CARTESIAN_POINT('Ctrl Pts',(7.04871331545306,218.809155844927,2.56944875671871));
#1761=CARTESIAN_POINT('Ctrl Pts',(6.99451296753855,218.74204613624,2.71813540129498));
#1762=CARTESIAN_POINT('Ctrl Pts',(6.93552054364113,218.674628800622,2.86533230206815));
#1763=CARTESIAN_POINT('Ctrl Pts',(6.87188471229629,218.607105531561,3.01058579312352));
#1764=CARTESIAN_POINT('Ctrl Pts',(6.81060403165534,218.542081286575,3.15046347852863));
#1765=CARTESIAN_POINT('Ctrl Pts',(6.7450177944479,218.476959054234,3.28853853492905));
#1766=CARTESIAN_POINT('Ctrl Pts',(6.6753084083992,218.411920847683,3.42442461876496));
#1767=CARTESIAN_POINT('Ctrl Pts',(6.60561114847611,218.346893954694,3.56028706486978));
#1768=CARTESIAN_POINT('Ctrl Pts',(6.53179244342414,218.281951283189,3.69396084347523));
#1769=CARTESIAN_POINT('Ctrl Pts',(6.45407988419915,218.217273190526,3.82508551083821));
#1770=CARTESIAN_POINT('Ctrl Pts',(6.3763464712596,218.152577741871,3.95624536474522));
#1771=CARTESIAN_POINT('Ctrl Pts',(6.29471745740002,218.088147231023,4.0848543388152));
#1772=CARTESIAN_POINT('Ctrl Pts',(6.20946132033851,218.02415727582,4.21058385833468));
#1773=CARTESIAN_POINT('Ctrl Pts',(6.19962572130945,218.016775056042,4.22508868089329));
#1774=CARTESIAN_POINT('Ctrl Pts',(6.18974188939196,218.009398692253,4.23955521930249));
#1775=CARTESIAN_POINT('Ctrl Pts',(6.17981026821525,218.002028447915,4.25398300016701));
#1776=CARTESIAN_POINT('Ctrl Pts',(6.09371831161196,217.938139708658,4.37904978050132));
#1777=CARTESIAN_POINT('Ctrl Pts',(6.00362010807817,217.87379055128,4.50180008775267));
#1778=CARTESIAN_POINT('Ctrl Pts',(5.9097213981558,217.809155844927,4.62186318631654));
#1779=CARTESIAN_POINT('Ctrl Pts',(5.81222710407562,217.742046136239,4.74652375992017));
#1780=CARTESIAN_POINT('Ctrl Pts',(5.71063563105773,217.674628800622,4.8682866700552));
#1781=CARTESIAN_POINT('Ctrl Pts',(5.605228561759,217.60710553156,4.98676639590123));
#1782=CARTESIAN_POINT('Ctrl Pts',(5.50372258918827,217.542081286575,5.10086120834527));
#1783=CARTESIAN_POINT('Ctrl Pts',(5.3986788319857,217.476959054234,5.21191112857863));
#1784=CARTESIAN_POINT('Ctrl Pts',(5.29039015693262,217.411920847682,5.31960508912823));
#1785=CARTESIAN_POINT('Ctrl Pts',(5.18212031897114,217.346893954693,5.42728031603836));
#1786=CARTESIAN_POINT('Ctrl Pts',(5.07060708921561,217.281951283188,5.53160039987501));
#1787=CARTESIAN_POINT('Ctrl Pts',(4.95617830276981,217.217273190525,5.63229286774066));
#1788=CARTESIAN_POINT('Ctrl Pts',(4.84171881002289,217.152577741871,5.73301235584603));
#1789=CARTESIAN_POINT('Ctrl Pts',(4.72434264585635,217.088147231022,5.83010200617252));
#1790=CARTESIAN_POINT('Ctrl Pts',(4.60440668292385,217.02415727582,5.92333228977531));
#1791=CARTESIAN_POINT('Ctrl Pts',(4.59057023570477,217.016775056041,5.9340878285374));
#1792=CARTESIAN_POINT('Ctrl Pts',(4.57669974673563,217.009398692253,5.94479205212752));
#1793=CARTESIAN_POINT('Ctrl Pts',(4.56279578422008,217.002028447915,5.95544464740896));
#1794=CARTESIAN_POINT('Ctrl Pts',(4.44226970733684,216.938139708657,6.04778634614857));
#1795=CARTESIAN_POINT('Ctrl Pts',(4.31864929275411,216.87379055128,6.13668694968261));
#1796=CARTESIAN_POINT('Ctrl Pts',(4.19224477495716,216.809155844927,6.22185744482248));
#1797=CARTESIAN_POINT('Ctrl Pts',(4.06099995549857,216.742046136239,6.31028930194794));
#1798=CARTESIAN_POINT('Ctrl Pts',(3.92675391456862,216.674628800622,6.3946992194288));
#1799=CARTESIAN_POINT('Ctrl Pts',(3.78989358567318,216.60710553156,6.47480755900296));
#1800=CARTESIAN_POINT('Ctrl Pts',(3.65809843300166,216.542081286575,6.55195110329844));
#1801=CARTESIAN_POINT('Ctrl Pts',(3.5238795706419,216.476959054234,6.62510554744185));
#1802=CARTESIAN_POINT('Ctrl Pts',(3.38761165659031,216.411920847682,6.69406554949845));
#1803=CARTESIAN_POINT('Ctrl Pts',(3.25136744669046,216.346893954693,6.76301355578654));
#1804=CARTESIAN_POINT('Ctrl Pts',(3.11307538411824,216.281951283188,6.82776836820773));
#1805=CARTESIAN_POINT('Ctrl Pts',(2.97313145734122,216.217273190525,6.88817215625573));
#1806=CARTESIAN_POINT('Ctrl Pts',(2.83314997742261,216.152577741871,6.94859215331013));
#1807=CARTESIAN_POINT('Ctrl Pts',(2.69151625970498,216.088147231022,7.00465866845613));
#1808=CARTESIAN_POINT('Ctrl Pts',(2.54864063859571,216.024157275819,7.0562636864099));
#1809=CARTESIAN_POINT('Ctrl Pts',(2.532157751045,216.016775056041,7.0622171143032));
#1810=CARTESIAN_POINT('Ctrl Pts',(2.51565834512628,216.009398692253,7.06811121908852));
#1811=CARTESIAN_POINT('Ctrl Pts',(2.49914305799789,216.002028447915,7.07394587853975));
#1812=CARTESIAN_POINT('Ctrl Pts',(2.35598079299496,215.938139708658,7.12452344682943));
#1813=CARTESIAN_POINT('Ctrl Pts',(2.2109389948571,215.87379055128,7.17087213616521));
#1814=CARTESIAN_POINT('Ctrl Pts',(2.0644020241,215.809155844927,7.21281294639896));
#1815=CARTESIAN_POINT('Ctrl Pts',(1.91225383662793,215.74204613624,7.25635976072988));
#1816=CARTESIAN_POINT('Ctrl Pts',(1.75849416561922,215.674628800623,7.29515405471512));
#1817=CARTESIAN_POINT('Ctrl Pts',(1.60357741968125,215.607105531561,7.32904944559231));
#1818=CARTESIAN_POINT('Ctrl Pts',(1.4543941147233,215.542081286575,7.3616903741329));
#1819=CARTESIAN_POINT('Ctrl Pts',(1.30413842461201,215.476959054234,7.38978847549662));
#1820=CARTESIAN_POINT('Ctrl Pts',(1.15323012442371,215.411920847683,7.41326423358633));
#1821=CARTESIAN_POINT('Ctrl Pts',(1.00234807511962,215.346893954693,7.43673590800796));
#1822=CARTESIAN_POINT('Ctrl Pts',(0.85081417035265,215.281951283189,7.45558679680064));
#1823=CARTESIAN_POINT('Ctrl Pts',(0.699053789843915,215.217273190525,7.46978916139897));
#1824=CARTESIAN_POINT('Ctrl Pts',(0.547252685316762,215.152577741871,7.4839953371195));
#1825=CARTESIAN_POINT('Ctrl Pts',(0.395225509158773,215.088147231022,7.49355053594384));
#1826=CARTESIAN_POINT('Ctrl Pts',(0.243395891140316,215.02415727582,7.49847882953767));
#1827=CARTESIAN_POINT('Ctrl Pts',(0.225880023133805,215.016775056041,7.49904738356035));
#1828=CARTESIAN_POINT('Ctrl Pts',(0.208366777074288,215.009398692253,7.49955441349819));
#1829=CARTESIAN_POINT('Ctrl Pts',(0.190856796705293,215.002028447915,7.5));
#1830=CARTESIAN_POINT('Ctrl Pts',(0.127311648028422,214.975281229334,7.50161706980302));
#1831=CARTESIAN_POINT('Ctrl Pts',(0.0636823578853861,214.948453397593,7.50242803155527));
#1832=CARTESIAN_POINT('Ctrl Pts',(-4.068439266928E-7,214.921557632927,7.50242802810187));
#1833=CARTESIAN_POINT('Origin',(0.190856796705285,235.002028447915,28.7581985010212));
#1834=CARTESIAN_POINT('',(0.190856796705285,235.002028447915,50.0163970020424));
#1835=CARTESIAN_POINT('Ctrl Pts',(0.190856796705285,235.002028447915,7.5));
#1836=CARTESIAN_POINT('Ctrl Pts',(0.190856796705285,235.002028447915,14.5858638315753));
#1837=CARTESIAN_POINT('Ctrl Pts',(0.190856796705285,235.002028447915,21.6717276631507));
#1838=CARTESIAN_POINT('Ctrl Pts',(0.190856796705285,235.002028447915,35.8438599971648));
#1839=CARTESIAN_POINT('Ctrl Pts',(0.190856796705285,235.002028447915,42.9301284996036));
#1840=CARTESIAN_POINT('Ctrl Pts',(0.190856796705285,235.002028447915,50.0163970020424));
#1841=CARTESIAN_POINT('',(0.000256710972400845,237.995967593475,50.0163970020424));
#1842=CARTESIAN_POINT('',(0.000256710972400879,237.995967593475,50.0163970020424));
#1843=CARTESIAN_POINT('',(0.190856796705286,235.002028447915,50.0163970020424));
#1844=CARTESIAN_POINT('Origin',(0.190856796705285,175.002028447915,28.7581985010212));
#1845=CARTESIAN_POINT('',(0.190856796705285,175.002028447915,50.0163970020424));
#1846=CARTESIAN_POINT('Ctrl Pts',(0.190856796705285,175.002028447915,50.0163970020424));
#1847=CARTESIAN_POINT('Ctrl Pts',(0.190856796705285,175.002028447915,42.9301284996036));
#1848=CARTESIAN_POINT('Ctrl Pts',(0.190856796705285,175.002028447915,35.8438599971648));
#1849=CARTESIAN_POINT('Ctrl Pts',(0.190856796705285,175.002028447915,21.6717276631507));
#1850=CARTESIAN_POINT('Ctrl Pts',(0.190856796705285,175.002028447915,14.5858638315753));
#1851=CARTESIAN_POINT('Ctrl Pts',(0.190856796705285,175.002028447915,7.5));
#1852=CARTESIAN_POINT('',(0.000256710972400845,177.995967593475,50.0163970020424));
#1853=CARTESIAN_POINT('',(0.000256710972401712,177.995967593475,50.0163970020424));
#1854=CARTESIAN_POINT('',(0.00025671097240121,177.995967593475,7.5));
#1855=CARTESIAN_POINT('Ctrl Pts',(0.190856796705285,235.002028447915,7.5));
#1856=CARTESIAN_POINT('Ctrl Pts',(-0.997026505728737,234.502028447915,7.5302287469283));
#1857=CARTESIAN_POINT('Ctrl Pts',(-2.13611185762632,234.002028447915,7.19190186588755));
#1858=CARTESIAN_POINT('Ctrl Pts',(-3.27519720952391,233.502028447915,6.8535749848468));
#1859=CARTESIAN_POINT('Ctrl Pts',(-4.25398300016701,233.002028447915,6.17981026821526));
#1860=CARTESIAN_POINT('Ctrl Pts',(-5.2327687908101,232.502028447915,5.50604555158371));
#1861=CARTESIAN_POINT('Ctrl Pts',(-5.95544464740896,232.002028447915,4.56279578422009));
#1862=CARTESIAN_POINT('Ctrl Pts',(-6.67812050400781,231.502028447915,3.61954601685647));
#1863=CARTESIAN_POINT('Ctrl Pts',(-7.07394587853975,231.002028447915,2.49914305799789));
#1864=CARTESIAN_POINT('Ctrl Pts',(-7.4697712530717,230.502028447915,1.37874009913931));
#1865=CARTESIAN_POINT('Ctrl Pts',(-7.5,230.002028447915,0.190856796705286));
#1866=CARTESIAN_POINT('Ctrl Pts',(-7.5302287469283,229.502028447915,-0.997026505728736));
#1867=CARTESIAN_POINT('Ctrl Pts',(-7.19190186588755,229.002028447915,-2.13611185762632));
#1868=CARTESIAN_POINT('Ctrl Pts',(-6.8535749848468,228.502028447915,-3.27519720952391));
#1869=CARTESIAN_POINT('Ctrl Pts',(-6.17981026821526,228.002028447915,-4.25398300016701));
#1870=CARTESIAN_POINT('Ctrl Pts',(-5.50604555158371,227.502028447915,-5.2327687908101));
#1871=CARTESIAN_POINT('Ctrl Pts',(-4.56279578422009,227.002028447915,-5.95544464740895));
#1872=CARTESIAN_POINT('Ctrl Pts',(-3.61954601685647,226.502028447915,-6.67812050400781));
#1873=CARTESIAN_POINT('Ctrl Pts',(-2.49914305799789,226.002028447915,-7.07394587853975));
#1874=CARTESIAN_POINT('Ctrl Pts',(-1.37874009913931,225.502028447915,-7.4697712530717));
#1875=CARTESIAN_POINT('Ctrl Pts',(-0.190856796705286,225.002028447915,-7.5));
#1876=CARTESIAN_POINT('Ctrl Pts',(0.997026505728736,224.502028447915,-7.5302287469283));
#1877=CARTESIAN_POINT('Ctrl Pts',(2.13611185762632,224.002028447915,-7.19190186588755));
#1878=CARTESIAN_POINT('Ctrl Pts',(3.27519720952391,223.502028447915,-6.8535749848468));
#1879=CARTESIAN_POINT('Ctrl Pts',(4.25398300016701,223.002028447915,-6.17981026821526));
#1880=CARTESIAN_POINT('Ctrl Pts',(5.2327687908101,222.502028447915,-5.50604555158371));
#1881=CARTESIAN_POINT('Ctrl Pts',(5.95544464740895,222.002028447915,-4.56279578422009));
#1882=CARTESIAN_POINT('Ctrl Pts',(6.67812050400781,221.502028447915,-3.61954601685647));
#1883=CARTESIAN_POINT('Ctrl Pts',(7.07394587853975,221.002028447915,-2.49914305799789));
#1884=CARTESIAN_POINT('Ctrl Pts',(7.4697712530717,220.502028447915,-1.37874009913931));
#1885=CARTESIAN_POINT('Ctrl Pts',(7.5,220.002028447915,-0.190856796705287));
#1886=CARTESIAN_POINT('Ctrl Pts',(7.5302287469283,219.502028447915,0.997026505728735));
#1887=CARTESIAN_POINT('Ctrl Pts',(7.19190186588755,219.002028447915,2.13611185762632));
#1888=CARTESIAN_POINT('Ctrl Pts',(6.8535749848468,218.502028447915,3.27519720952391));
#1889=CARTESIAN_POINT('Ctrl Pts',(6.17981026821526,218.002028447915,4.25398300016701));
#1890=CARTESIAN_POINT('Ctrl Pts',(5.50604555158371,217.502028447915,5.2327687908101));
#1891=CARTESIAN_POINT('Ctrl Pts',(4.56279578422009,217.002028447915,5.95544464740895));
#1892=CARTESIAN_POINT('Ctrl Pts',(3.61954601685647,216.502028447915,6.67812050400781));
#1893=CARTESIAN_POINT('Ctrl Pts',(2.49914305799789,216.002028447915,7.07394587853975));
#1894=CARTESIAN_POINT('Ctrl Pts',(1.37874009913931,215.502028447915,7.4697712530717));
#1895=CARTESIAN_POINT('Ctrl Pts',(0.190856796705285,215.002028447915,7.5));
#1896=CARTESIAN_POINT('Ctrl Pts',(-0.997026505728737,214.502028447915,7.5302287469283));
#1897=CARTESIAN_POINT('Ctrl Pts',(-2.13611185762632,214.002028447915,7.19190186588755));
#1898=CARTESIAN_POINT('Ctrl Pts',(-3.27519720952391,213.502028447915,6.8535749848468));
#1899=CARTESIAN_POINT('Ctrl Pts',(-4.25398300016701,213.002028447915,6.17981026821526));
#1900=CARTESIAN_POINT('Ctrl Pts',(-5.2327687908101,212.502028447915,5.50604555158371));
#1901=CARTESIAN_POINT('Ctrl Pts',(-5.95544464740896,212.002028447915,4.56279578422009));
#1902=CARTESIAN_POINT('Ctrl Pts',(-6.67812050400781,211.502028447915,3.61954601685647));
#1903=CARTESIAN_POINT('Ctrl Pts',(-7.07394587853975,211.002028447915,2.49914305799789));
#1904=CARTESIAN_POINT('Ctrl Pts',(-7.4697712530717,210.502028447915,1.37874009913931));
#1905=CARTESIAN_POINT('Ctrl Pts',(-7.5,210.002028447915,0.190856796705286));
#1906=CARTESIAN_POINT('Ctrl Pts',(-7.5302287469283,209.502028447915,-0.997026505728736));
#1907=CARTESIAN_POINT('Ctrl Pts',(-7.19190186588755,209.002028447915,-2.13611185762632));
#1908=CARTESIAN_POINT('Ctrl Pts',(-6.8535749848468,208.502028447915,-3.27519720952391));
#1909=CARTESIAN_POINT('Ctrl Pts',(-6.17981026821526,208.002028447915,-4.25398300016701));
#1910=CARTESIAN_POINT('Ctrl Pts',(-5.50604555158371,207.502028447915,-5.2327687908101));
#1911=CARTESIAN_POINT('Ctrl Pts',(-4.56279578422009,207.002028447915,-5.95544464740895));
#1912=CARTESIAN_POINT('Ctrl Pts',(-3.61954601685647,206.502028447915,-6.67812050400781));
#1913=CARTESIAN_POINT('Ctrl Pts',(-2.49914305799789,206.002028447915,-7.07394587853975));
#1914=CARTESIAN_POINT('Ctrl Pts',(-1.37874009913931,205.502028447915,-7.4697712530717));
#1915=CARTESIAN_POINT('Ctrl Pts',(-0.190856796705286,205.002028447915,-7.5));
#1916=CARTESIAN_POINT('Ctrl Pts',(0.997026505728736,204.502028447915,-7.5302287469283));
#1917=CARTESIAN_POINT('Ctrl Pts',(2.13611185762632,204.002028447915,-7.19190186588755));
#1918=CARTESIAN_POINT('Ctrl Pts',(3.27519720952391,203.502028447915,-6.8535749848468));
#1919=CARTESIAN_POINT('Ctrl Pts',(4.25398300016701,203.002028447915,-6.17981026821526));
#1920=CARTESIAN_POINT('Ctrl Pts',(5.2327687908101,202.502028447915,-5.50604555158371));
#1921=CARTESIAN_POINT('Ctrl Pts',(5.95544464740895,202.002028447915,-4.56279578422009));
#1922=CARTESIAN_POINT('Ctrl Pts',(6.67812050400781,201.502028447915,-3.61954601685647));
#1923=CARTESIAN_POINT('Ctrl Pts',(7.07394587853975,201.002028447915,-2.49914305799789));
#1924=CARTESIAN_POINT('Ctrl Pts',(7.4697712530717,200.502028447915,-1.37874009913931));
#1925=CARTESIAN_POINT('Ctrl Pts',(7.5,200.002028447915,-0.190856796705287));
#1926=CARTESIAN_POINT('Ctrl Pts',(7.5302287469283,199.502028447915,0.997026505728735));
#1927=CARTESIAN_POINT('Ctrl Pts',(7.19190186588755,199.002028447915,2.13611185762632));
#1928=CARTESIAN_POINT('Ctrl Pts',(6.8535749848468,198.502028447915,3.27519720952391));
#1929=CARTESIAN_POINT('Ctrl Pts',(6.17981026821526,198.002028447915,4.25398300016701));
#1930=CARTESIAN_POINT('Ctrl Pts',(5.50604555158371,197.502028447915,5.2327687908101));
#1931=CARTESIAN_POINT('Ctrl Pts',(4.56279578422009,197.002028447915,5.95544464740895));
#1932=CARTESIAN_POINT('Ctrl Pts',(3.61954601685647,196.502028447915,6.67812050400781));
#1933=CARTESIAN_POINT('Ctrl Pts',(2.49914305799789,196.002028447915,7.07394587853975));
#1934=CARTESIAN_POINT('Ctrl Pts',(1.37874009913931,195.502028447915,7.4697712530717));
#1935=CARTESIAN_POINT('Ctrl Pts',(0.190856796705285,195.002028447915,7.5));
#1936=CARTESIAN_POINT('Ctrl Pts',(-0.997026505728737,194.502028447915,7.5302287469283));
#1937=CARTESIAN_POINT('Ctrl Pts',(-2.13611185762632,194.002028447915,7.19190186588755));
#1938=CARTESIAN_POINT('Ctrl Pts',(-3.27519720952391,193.502028447915,6.8535749848468));
#1939=CARTESIAN_POINT('Ctrl Pts',(-4.25398300016701,193.002028447915,6.17981026821526));
#1940=CARTESIAN_POINT('Ctrl Pts',(-5.2327687908101,192.502028447915,5.50604555158371));
#1941=CARTESIAN_POINT('Ctrl Pts',(-5.95544464740896,192.002028447915,4.56279578422009));
#1942=CARTESIAN_POINT('Ctrl Pts',(-6.67812050400781,191.502028447915,3.61954601685647));
#1943=CARTESIAN_POINT('Ctrl Pts',(-7.07394587853975,191.002028447915,2.49914305799789));
#1944=CARTESIAN_POINT('Ctrl Pts',(-7.4697712530717,190.502028447915,1.37874009913931));
#1945=CARTESIAN_POINT('Ctrl Pts',(-7.5,190.002028447915,0.190856796705286));
#1946=CARTESIAN_POINT('Ctrl Pts',(-7.5302287469283,189.502028447915,-0.997026505728736));
#1947=CARTESIAN_POINT('Ctrl Pts',(-7.19190186588755,189.002028447915,-2.13611185762632));
#1948=CARTESIAN_POINT('Ctrl Pts',(-6.8535749848468,188.502028447915,-3.27519720952391));
#1949=CARTESIAN_POINT('Ctrl Pts',(-6.17981026821526,188.002028447915,-4.25398300016701));
#1950=CARTESIAN_POINT('Ctrl Pts',(-5.50604555158371,187.502028447915,-5.2327687908101));
#1951=CARTESIAN_POINT('Ctrl Pts',(-4.56279578422009,187.002028447915,-5.95544464740895));
#1952=CARTESIAN_POINT('Ctrl Pts',(-3.61954601685647,186.502028447915,-6.67812050400781));
#1953=CARTESIAN_POINT('Ctrl Pts',(-2.49914305799789,186.002028447915,-7.07394587853975));
#1954=CARTESIAN_POINT('Ctrl Pts',(-1.37874009913931,185.502028447915,-7.4697712530717));
#1955=CARTESIAN_POINT('Ctrl Pts',(-0.190856796705286,185.002028447915,-7.5));
#1956=CARTESIAN_POINT('Ctrl Pts',(0.997026505728736,184.502028447915,-7.5302287469283));
#1957=CARTESIAN_POINT('Ctrl Pts',(2.13611185762632,184.002028447915,-7.19190186588755));
#1958=CARTESIAN_POINT('Ctrl Pts',(3.27519720952391,183.502028447915,-6.8535749848468));
#1959=CARTESIAN_POINT('Ctrl Pts',(4.25398300016701,183.002028447915,-6.17981026821526));
#1960=CARTESIAN_POINT('Ctrl Pts',(5.2327687908101,182.502028447915,-5.50604555158371));
#1961=CARTESIAN_POINT('Ctrl Pts',(5.95544464740895,182.002028447915,-4.56279578422009));
#1962=CARTESIAN_POINT('Ctrl Pts',(6.67812050400781,181.502028447915,-3.61954601685647));
#1963=CARTESIAN_POINT('Ctrl Pts',(7.07394587853975,181.002028447915,-2.49914305799789));
#1964=CARTESIAN_POINT('Ctrl Pts',(7.4697712530717,180.502028447915,-1.37874009913931));
#1965=CARTESIAN_POINT('Ctrl Pts',(7.5,180.002028447915,-0.190856796705287));
#1966=CARTESIAN_POINT('Ctrl Pts',(7.5302287469283,179.502028447915,0.997026505728735));
#1967=CARTESIAN_POINT('Ctrl Pts',(7.19190186588755,179.002028447915,2.13611185762632));
#1968=CARTESIAN_POINT('Ctrl Pts',(6.8535749848468,178.502028447915,3.27519720952391));
#1969=CARTESIAN_POINT('Ctrl Pts',(6.17981026821526,178.002028447915,4.25398300016701));
#1970=CARTESIAN_POINT('Ctrl Pts',(5.50604555158371,177.502028447915,5.2327687908101));
#1971=CARTESIAN_POINT('Ctrl Pts',(4.56279578422009,177.002028447915,5.95544464740895));
#1972=CARTESIAN_POINT('Ctrl Pts',(3.61954601685647,176.502028447915,6.67812050400781));
#1973=CARTESIAN_POINT('Ctrl Pts',(2.49914305799789,176.002028447915,7.07394587853975));
#1974=CARTESIAN_POINT('Ctrl Pts',(1.37874009913931,175.502028447915,7.4697712530717));
#1975=CARTESIAN_POINT('Ctrl Pts',(0.190856796705285,175.002028447915,7.5));
#1976=CARTESIAN_POINT('Ctrl Pts',(0.190856796705285,235.002028447915,50.0163970020424));
#1977=CARTESIAN_POINT('Ctrl Pts',(-7.73096224951301,234.502028447915,50.0466257489707));
#1978=CARTESIAN_POINT('Ctrl Pts',(-15.2744010708495,234.002028447915,47.6273982840717));
#1979=CARTESIAN_POINT('Ctrl Pts',(-22.817839892186,233.502028447915,45.2081708191727));
#1980=CARTESIAN_POINT('Ctrl Pts',(-29.2444941385794,233.002028447915,40.5762979824596));
#1981=CARTESIAN_POINT('Ctrl Pts',(-35.6711483849729,232.502028447915,35.9444251457465));
#1982=CARTESIAN_POINT('Ctrl Pts',(-40.3519323616533,232.002028447915,29.5533069226325));
#1983=CARTESIAN_POINT('Ctrl Pts',(-45.0327163383337,231.502028447915,23.1621886995185));
#1984=CARTESIAN_POINT('Ctrl Pts',(-47.5094422967239,231.002028447915,15.6374322712211));
#1985=CARTESIAN_POINT('Ctrl Pts',(-49.9861682551141,230.502028447915,8.11267584292358));
#1986=CARTESIAN_POINT('Ctrl Pts',(-50.0163970020424,230.002028447915,0.190856796705288));
#1987=CARTESIAN_POINT('Ctrl Pts',(-50.0466257489707,229.502028447915,-7.73096224951301));
#1988=CARTESIAN_POINT('Ctrl Pts',(-47.6273982840717,229.002028447915,-15.2744010708495));
#1989=CARTESIAN_POINT('Ctrl Pts',(-45.2081708191727,228.502028447915,-22.817839892186));
#1990=CARTESIAN_POINT('Ctrl Pts',(-40.5762979824596,228.002028447915,-29.2444941385794));
#1991=CARTESIAN_POINT('Ctrl Pts',(-35.9444251457465,227.502028447915,-35.6711483849729));
#1992=CARTESIAN_POINT('Ctrl Pts',(-29.5533069226325,227.002028447915,-40.3519323616533));
#1993=CARTESIAN_POINT('Ctrl Pts',(-23.1621886995185,226.502028447915,-45.0327163383337));
#1994=CARTESIAN_POINT('Ctrl Pts',(-15.6374322712211,226.002028447915,-47.5094422967239));
#1995=CARTESIAN_POINT('Ctrl Pts',(-8.11267584292359,225.502028447915,-49.9861682551141));
#1996=CARTESIAN_POINT('Ctrl Pts',(-0.190856796705292,225.002028447915,-50.0163970020424));
#1997=CARTESIAN_POINT('Ctrl Pts',(7.730962249513,224.502028447915,-50.0466257489707));
#1998=CARTESIAN_POINT('Ctrl Pts',(15.2744010708495,224.002028447915,-47.6273982840717));
#1999=CARTESIAN_POINT('Ctrl Pts',(22.817839892186,223.502028447915,-45.2081708191727));
#2000=CARTESIAN_POINT('Ctrl Pts',(29.2444941385794,223.002028447915,-40.5762979824596));
#2001=CARTESIAN_POINT('Ctrl Pts',(35.6711483849729,222.502028447915,-35.9444251457465));
#2002=CARTESIAN_POINT('Ctrl Pts',(40.3519323616533,222.002028447915,-29.5533069226325));
#2003=CARTESIAN_POINT('Ctrl Pts',(45.0327163383337,221.502028447915,-23.1621886995185));
#2004=CARTESIAN_POINT('Ctrl Pts',(47.5094422967239,221.002028447915,-15.6374322712211));
#2005=CARTESIAN_POINT('Ctrl Pts',(49.9861682551141,220.502028447915,-8.11267584292359));
#2006=CARTESIAN_POINT('Ctrl Pts',(50.0163970020424,220.002028447915,-0.190856796705295));
#2007=CARTESIAN_POINT('Ctrl Pts',(50.0466257489707,219.502028447915,7.730962249513));
#2008=CARTESIAN_POINT('Ctrl Pts',(47.6273982840717,219.002028447915,15.2744010708495));
#2009=CARTESIAN_POINT('Ctrl Pts',(45.2081708191727,218.502028447915,22.817839892186));
#2010=CARTESIAN_POINT('Ctrl Pts',(40.5762979824596,218.002028447915,29.2444941385794));
#2011=CARTESIAN_POINT('Ctrl Pts',(35.9444251457465,217.502028447915,35.6711483849729));
#2012=CARTESIAN_POINT('Ctrl Pts',(29.5533069226325,217.002028447915,40.3519323616533));
#2013=CARTESIAN_POINT('Ctrl Pts',(23.1621886995185,216.502028447915,45.0327163383337));
#2014=CARTESIAN_POINT('Ctrl Pts',(15.6374322712211,216.002028447915,47.5094422967239));
#2015=CARTESIAN_POINT('Ctrl Pts',(8.11267584292359,215.502028447915,49.9861682551141));
#2016=CARTESIAN_POINT('Ctrl Pts',(0.190856796705285,215.002028447915,50.0163970020424));
#2017=CARTESIAN_POINT('Ctrl Pts',(-7.73096224951301,214.502028447915,50.0466257489707));
#2018=CARTESIAN_POINT('Ctrl Pts',(-15.2744010708495,214.002028447915,47.6273982840717));
#2019=CARTESIAN_POINT('Ctrl Pts',(-22.817839892186,213.502028447915,45.2081708191727));
#2020=CARTESIAN_POINT('Ctrl Pts',(-29.2444941385794,213.002028447915,40.5762979824596));
#2021=CARTESIAN_POINT('Ctrl Pts',(-35.6711483849729,212.502028447915,35.9444251457465));
#2022=CARTESIAN_POINT('Ctrl Pts',(-40.3519323616533,212.002028447915,29.5533069226325));
#2023=CARTESIAN_POINT('Ctrl Pts',(-45.0327163383337,211.502028447915,23.1621886995185));
#2024=CARTESIAN_POINT('Ctrl Pts',(-47.5094422967239,211.002028447915,15.6374322712211));
#2025=CARTESIAN_POINT('Ctrl Pts',(-49.9861682551141,210.502028447915,8.11267584292358));
#2026=CARTESIAN_POINT('Ctrl Pts',(-50.0163970020424,210.002028447915,0.190856796705288));
#2027=CARTESIAN_POINT('Ctrl Pts',(-50.0466257489707,209.502028447915,-7.73096224951301));
#2028=CARTESIAN_POINT('Ctrl Pts',(-47.6273982840717,209.002028447915,-15.2744010708495));
#2029=CARTESIAN_POINT('Ctrl Pts',(-45.2081708191727,208.502028447915,-22.817839892186));
#2030=CARTESIAN_POINT('Ctrl Pts',(-40.5762979824596,208.002028447915,-29.2444941385794));
#2031=CARTESIAN_POINT('Ctrl Pts',(-35.9444251457465,207.502028447915,-35.6711483849729));
#2032=CARTESIAN_POINT('Ctrl Pts',(-29.5533069226325,207.002028447915,-40.3519323616533));
#2033=CARTESIAN_POINT('Ctrl Pts',(-23.1621886995185,206.502028447915,-45.0327163383337));
#2034=CARTESIAN_POINT('Ctrl Pts',(-15.6374322712211,206.002028447915,-47.5094422967239));
#2035=CARTESIAN_POINT('Ctrl Pts',(-8.11267584292359,205.502028447915,-49.9861682551141));
#2036=CARTESIAN_POINT('Ctrl Pts',(-0.190856796705292,205.002028447915,-50.0163970020424));
#2037=CARTESIAN_POINT('Ctrl Pts',(7.730962249513,204.502028447915,-50.0466257489707));
#2038=CARTESIAN_POINT('Ctrl Pts',(15.2744010708495,204.002028447915,-47.6273982840717));
#2039=CARTESIAN_POINT('Ctrl Pts',(22.817839892186,203.502028447915,-45.2081708191727));
#2040=CARTESIAN_POINT('Ctrl Pts',(29.2444941385794,203.002028447915,-40.5762979824596));
#2041=CARTESIAN_POINT('Ctrl Pts',(35.6711483849729,202.502028447915,-35.9444251457465));
#2042=CARTESIAN_POINT('Ctrl Pts',(40.3519323616533,202.002028447915,-29.5533069226325));
#2043=CARTESIAN_POINT('Ctrl Pts',(45.0327163383337,201.502028447915,-23.1621886995185));
#2044=CARTESIAN_POINT('Ctrl Pts',(47.5094422967239,201.002028447915,-15.6374322712211));
#2045=CARTESIAN_POINT('Ctrl Pts',(49.9861682551141,200.502028447915,-8.11267584292359));
#2046=CARTESIAN_POINT('Ctrl Pts',(50.0163970020424,200.002028447915,-0.190856796705295));
#2047=CARTESIAN_POINT('Ctrl Pts',(50.0466257489707,199.502028447915,7.730962249513));
#2048=CARTESIAN_POINT('Ctrl Pts',(47.6273982840717,199.002028447915,15.2744010708495));
#2049=CARTESIAN_POINT('Ctrl Pts',(45.2081708191727,198.502028447915,22.817839892186));
#2050=CARTESIAN_POINT('Ctrl Pts',(40.5762979824596,198.002028447915,29.2444941385794));
#2051=CARTESIAN_POINT('Ctrl Pts',(35.9444251457465,197.502028447915,35.6711483849729));
#2052=CARTESIAN_POINT('Ctrl Pts',(29.5533069226325,197.002028447915,40.3519323616533));
#2053=CARTESIAN_POINT('Ctrl Pts',(23.1621886995185,196.502028447915,45.0327163383337));
#2054=CARTESIAN_POINT('Ctrl Pts',(15.6374322712211,196.002028447915,47.5094422967239));
#2055=CARTESIAN_POINT('Ctrl Pts',(8.11267584292359,195.502028447915,49.9861682551141));
#2056=CARTESIAN_POINT('Ctrl Pts',(0.190856796705285,195.002028447915,50.0163970020424));
#2057=CARTESIAN_POINT('Ctrl Pts',(-7.73096224951301,194.502028447915,50.0466257489707));
#2058=CARTESIAN_POINT('Ctrl Pts',(-15.2744010708495,194.002028447915,47.6273982840717));
#2059=CARTESIAN_POINT('Ctrl Pts',(-22.817839892186,193.502028447915,45.2081708191727));
#2060=CARTESIAN_POINT('Ctrl Pts',(-29.2444941385794,193.002028447915,40.5762979824596));
#2061=CARTESIAN_POINT('Ctrl Pts',(-35.6711483849729,192.502028447915,35.9444251457465));
#2062=CARTESIAN_POINT('Ctrl Pts',(-40.3519323616533,192.002028447915,29.5533069226325));
#2063=CARTESIAN_POINT('Ctrl Pts',(-45.0327163383337,191.502028447915,23.1621886995185));
#2064=CARTESIAN_POINT('Ctrl Pts',(-47.5094422967239,191.002028447915,15.6374322712211));
#2065=CARTESIAN_POINT('Ctrl Pts',(-49.9861682551141,190.502028447915,8.11267584292358));
#2066=CARTESIAN_POINT('Ctrl Pts',(-50.0163970020424,190.002028447915,0.190856796705288));
#2067=CARTESIAN_POINT('Ctrl Pts',(-50.0466257489707,189.502028447915,-7.73096224951301));
#2068=CARTESIAN_POINT('Ctrl Pts',(-47.6273982840717,189.002028447915,-15.2744010708495));
#2069=CARTESIAN_POINT('Ctrl Pts',(-45.2081708191727,188.502028447915,-22.817839892186));
#2070=CARTESIAN_POINT('Ctrl Pts',(-40.5762979824596,188.002028447915,-29.2444941385794));
#2071=CARTESIAN_POINT('Ctrl Pts',(-35.9444251457465,187.502028447915,-35.6711483849729));
#2072=CARTESIAN_POINT('Ctrl Pts',(-29.5533069226325,187.002028447915,-40.3519323616533));
#2073=CARTESIAN_POINT('Ctrl Pts',(-23.1621886995185,186.502028447915,-45.0327163383337));
#2074=CARTESIAN_POINT('Ctrl Pts',(-15.6374322712211,186.002028447915,-47.5094422967239));
#2075=CARTESIAN_POINT('Ctrl Pts',(-8.11267584292359,185.502028447915,-49.9861682551141));
#2076=CARTESIAN_POINT('Ctrl Pts',(-0.190856796705292,185.002028447915,-50.0163970020424));
#2077=CARTESIAN_POINT('Ctrl Pts',(7.730962249513,184.502028447915,-50.0466257489707));
#2078=CARTESIAN_POINT('Ctrl Pts',(15.2744010708495,184.002028447915,-47.6273982840717));
#2079=CARTESIAN_POINT('Ctrl Pts',(22.817839892186,183.502028447915,-45.2081708191727));
#2080=CARTESIAN_POINT('Ctrl Pts',(29.2444941385794,183.002028447915,-40.5762979824596));
#2081=CARTESIAN_POINT('Ctrl Pts',(35.6711483849729,182.502028447915,-35.9444251457465));
#2082=CARTESIAN_POINT('Ctrl Pts',(40.3519323616533,182.002028447915,-29.5533069226325));
#2083=CARTESIAN_POINT('Ctrl Pts',(45.0327163383337,181.502028447915,-23.1621886995185));
#2084=CARTESIAN_POINT('Ctrl Pts',(47.5094422967239,181.002028447915,-15.6374322712211));
#2085=CARTESIAN_POINT('Ctrl Pts',(49.9861682551141,180.502028447915,-8.11267584292359));
#2086=CARTESIAN_POINT('Ctrl Pts',(50.0163970020424,180.002028447915,-0.190856796705295));
#2087=CARTESIAN_POINT('Ctrl Pts',(50.0466257489707,179.502028447915,7.730962249513));
#2088=CARTESIAN_POINT('Ctrl Pts',(47.6273982840717,179.002028447915,15.2744010708495));
#2089=CARTESIAN_POINT('Ctrl Pts',(45.2081708191727,178.502028447915,22.817839892186));
#2090=CARTESIAN_POINT('Ctrl Pts',(40.5762979824596,178.002028447915,29.2444941385794));
#2091=CARTESIAN_POINT('Ctrl Pts',(35.9444251457465,177.502028447915,35.6711483849729));
#2092=CARTESIAN_POINT('Ctrl Pts',(29.5533069226325,177.002028447915,40.3519323616533));
#2093=CARTESIAN_POINT('Ctrl Pts',(23.1621886995185,176.502028447915,45.0327163383337));
#2094=CARTESIAN_POINT('Ctrl Pts',(15.6374322712211,176.002028447915,47.5094422967239));
#2095=CARTESIAN_POINT('Ctrl Pts',(8.11267584292359,175.502028447915,49.9861682551141));
#2096=CARTESIAN_POINT('Ctrl Pts',(0.190856796705285,175.002028447915,50.0163970020424));
#2097=CARTESIAN_POINT('Ctrl Pts',(0.190856796705285,235.002028447915,50.0163970020424));
#2098=CARTESIAN_POINT('Ctrl Pts',(-7.73096224951301,234.502028447915,50.0466257489707));
#2099=CARTESIAN_POINT('Ctrl Pts',(-15.2744010708495,234.002028447915,47.6273982840717));
#2100=CARTESIAN_POINT('Ctrl Pts',(-22.817839892186,233.502028447915,45.2081708191727));
#2101=CARTESIAN_POINT('Ctrl Pts',(-29.2444941385794,233.002028447915,40.5762979824596));
#2102=CARTESIAN_POINT('Ctrl Pts',(-35.6711483849729,232.502028447915,35.9444251457465));
#2103=CARTESIAN_POINT('Ctrl Pts',(-40.3519323616533,232.002028447915,29.5533069226325));
#2104=CARTESIAN_POINT('Ctrl Pts',(-45.0327163383337,231.502028447915,23.1621886995185));
#2105=CARTESIAN_POINT('Ctrl Pts',(-47.5094422967239,231.002028447915,15.6374322712211));
#2106=CARTESIAN_POINT('Ctrl Pts',(-49.9861682551141,230.502028447915,8.11267584292358));
#2107=CARTESIAN_POINT('Ctrl Pts',(-50.0163970020424,230.002028447915,0.190856796705288));
#2108=CARTESIAN_POINT('Ctrl Pts',(-50.0466257489707,229.502028447915,-7.73096224951301));
#2109=CARTESIAN_POINT('Ctrl Pts',(-47.6273982840717,229.002028447915,-15.2744010708495));
#2110=CARTESIAN_POINT('Ctrl Pts',(-45.2081708191727,228.502028447915,-22.817839892186));
#2111=CARTESIAN_POINT('Ctrl Pts',(-40.5762979824596,228.002028447915,-29.2444941385794));
#2112=CARTESIAN_POINT('Ctrl Pts',(-35.9444251457465,227.502028447915,-35.6711483849729));
#2113=CARTESIAN_POINT('Ctrl Pts',(-29.5533069226325,227.002028447915,-40.3519323616533));
#2114=CARTESIAN_POINT('Ctrl Pts',(-23.1621886995185,226.502028447915,-45.0327163383337));
#2115=CARTESIAN_POINT('Ctrl Pts',(-15.6374322712211,226.002028447915,-47.5094422967239));
#2116=CARTESIAN_POINT('Ctrl Pts',(-8.11267584292359,225.502028447915,-49.9861682551141));
#2117=CARTESIAN_POINT('Ctrl Pts',(-0.190856796705292,225.002028447915,-50.0163970020424));
#2118=CARTESIAN_POINT('Ctrl Pts',(7.730962249513,224.502028447915,-50.0466257489707));
#2119=CARTESIAN_POINT('Ctrl Pts',(15.2744010708495,224.002028447915,-47.6273982840717));
#2120=CARTESIAN_POINT('Ctrl Pts',(22.817839892186,223.502028447915,-45.2081708191727));
#2121=CARTESIAN_POINT('Ctrl Pts',(29.2444941385794,223.002028447915,-40.5762979824596));
#2122=CARTESIAN_POINT('Ctrl Pts',(35.6711483849729,222.502028447915,-35.9444251457465));
#2123=CARTESIAN_POINT('Ctrl Pts',(40.3519323616533,222.002028447915,-29.5533069226325));
#2124=CARTESIAN_POINT('Ctrl Pts',(45.0327163383337,221.502028447915,-23.1621886995185));
#2125=CARTESIAN_POINT('Ctrl Pts',(47.5094422967239,221.002028447915,-15.6374322712211));
#2126=CARTESIAN_POINT('Ctrl Pts',(49.9861682551141,220.502028447915,-8.11267584292359));
#2127=CARTESIAN_POINT('Ctrl Pts',(50.0163970020424,220.002028447915,-0.190856796705295));
#2128=CARTESIAN_POINT('Ctrl Pts',(50.0466257489707,219.502028447915,7.730962249513));
#2129=CARTESIAN_POINT('Ctrl Pts',(47.6273982840717,219.002028447915,15.2744010708495));
#2130=CARTESIAN_POINT('Ctrl Pts',(45.2081708191727,218.502028447915,22.817839892186));
#2131=CARTESIAN_POINT('Ctrl Pts',(40.5762979824596,218.002028447915,29.2444941385794));
#2132=CARTESIAN_POINT('Ctrl Pts',(35.9444251457465,217.502028447915,35.6711483849729));
#2133=CARTESIAN_POINT('Ctrl Pts',(29.5533069226325,217.002028447915,40.3519323616533));
#2134=CARTESIAN_POINT('Ctrl Pts',(23.1621886995185,216.502028447915,45.0327163383337));
#2135=CARTESIAN_POINT('Ctrl Pts',(15.6374322712211,216.002028447915,47.5094422967239));
#2136=CARTESIAN_POINT('Ctrl Pts',(8.11267584292359,215.502028447915,49.9861682551141));
#2137=CARTESIAN_POINT('Ctrl Pts',(0.190856796705285,215.002028447915,50.0163970020424));
#2138=CARTESIAN_POINT('Ctrl Pts',(-7.73096224951301,214.502028447915,50.0466257489707));
#2139=CARTESIAN_POINT('Ctrl Pts',(-15.2744010708495,214.002028447915,47.6273982840717));
#2140=CARTESIAN_POINT('Ctrl Pts',(-22.817839892186,213.502028447915,45.2081708191727));
#2141=CARTESIAN_POINT('Ctrl Pts',(-29.2444941385794,213.002028447915,40.5762979824596));
#2142=CARTESIAN_POINT('Ctrl Pts',(-35.6711483849729,212.502028447915,35.9444251457465));
#2143=CARTESIAN_POINT('Ctrl Pts',(-40.3519323616533,212.002028447915,29.5533069226325));
#2144=CARTESIAN_POINT('Ctrl Pts',(-45.0327163383337,211.502028447915,23.1621886995185));
#2145=CARTESIAN_POINT('Ctrl Pts',(-47.5094422967239,211.002028447915,15.6374322712211));
#2146=CARTESIAN_POINT('Ctrl Pts',(-49.9861682551141,210.502028447915,8.11267584292358));
#2147=CARTESIAN_POINT('Ctrl Pts',(-50.0163970020424,210.002028447915,0.190856796705288));
#2148=CARTESIAN_POINT('Ctrl Pts',(-50.0466257489707,209.502028447915,-7.73096224951301));
#2149=CARTESIAN_POINT('Ctrl Pts',(-47.6273982840717,209.002028447915,-15.2744010708495));
#2150=CARTESIAN_POINT('Ctrl Pts',(-45.2081708191727,208.502028447915,-22.817839892186));
#2151=CARTESIAN_POINT('Ctrl Pts',(-40.5762979824596,208.002028447915,-29.2444941385794));
#2152=CARTESIAN_POINT('Ctrl Pts',(-35.9444251457465,207.502028447915,-35.6711483849729));
#2153=CARTESIAN_POINT('Ctrl Pts',(-29.5533069226325,207.002028447915,-40.3519323616533));
#2154=CARTESIAN_POINT('Ctrl Pts',(-23.1621886995185,206.502028447915,-45.0327163383337));
#2155=CARTESIAN_POINT('Ctrl Pts',(-15.6374322712211,206.002028447915,-47.5094422967239));
#2156=CARTESIAN_POINT('Ctrl Pts',(-8.11267584292359,205.502028447915,-49.9861682551141));
#2157=CARTESIAN_POINT('Ctrl Pts',(-0.190856796705292,205.002028447915,-50.0163970020424));
#2158=CARTESIAN_POINT('Ctrl Pts',(7.730962249513,204.502028447915,-50.0466257489707));
#2159=CARTESIAN_POINT('Ctrl Pts',(15.2744010708495,204.002028447915,-47.6273982840717));
#2160=CARTESIAN_POINT('Ctrl Pts',(22.817839892186,203.502028447915,-45.2081708191727));
#2161=CARTESIAN_POINT('Ctrl Pts',(29.2444941385794,203.002028447915,-40.5762979824596));
#2162=CARTESIAN_POINT('Ctrl Pts',(35.6711483849729,202.502028447915,-35.9444251457465));
#2163=CARTESIAN_POINT('Ctrl Pts',(40.3519323616533,202.002028447915,-29.5533069226325));
#2164=CARTESIAN_POINT('Ctrl Pts',(45.0327163383337,201.502028447915,-23.1621886995185));
#2165=CARTESIAN_POINT('Ctrl Pts',(47.5094422967239,201.002028447915,-15.6374322712211));
#2166=CARTESIAN_POINT('Ctrl Pts',(49.9861682551141,200.502028447915,-8.11267584292359));
#2167=CARTESIAN_POINT('Ctrl Pts',(50.0163970020424,200.002028447915,-0.190856796705295));
#2168=CARTESIAN_POINT('Ctrl Pts',(50.0466257489707,199.502028447915,7.730962249513));
#2169=CARTESIAN_POINT('Ctrl Pts',(47.6273982840717,199.002028447915,15.2744010708495));
#2170=CARTESIAN_POINT('Ctrl Pts',(45.2081708191727,198.502028447915,22.817839892186));
#2171=CARTESIAN_POINT('Ctrl Pts',(40.5762979824596,198.002028447915,29.2444941385794));
#2172=CARTESIAN_POINT('Ctrl Pts',(35.9444251457465,197.502028447915,35.6711483849729));
#2173=CARTESIAN_POINT('Ctrl Pts',(29.5533069226325,197.002028447915,40.3519323616533));
#2174=CARTESIAN_POINT('Ctrl Pts',(23.1621886995185,196.502028447915,45.0327163383337));
#2175=CARTESIAN_POINT('Ctrl Pts',(15.6374322712211,196.002028447915,47.5094422967239));
#2176=CARTESIAN_POINT('Ctrl Pts',(8.11267584292359,195.502028447915,49.9861682551141));
#2177=CARTESIAN_POINT('Ctrl Pts',(0.190856796705285,195.002028447915,50.0163970020424));
#2178=CARTESIAN_POINT('Ctrl Pts',(-7.73096224951301,194.502028447915,50.0466257489707));
#2179=CARTESIAN_POINT('Ctrl Pts',(-15.2744010708495,194.002028447915,47.6273982840717));
#2180=CARTESIAN_POINT('Ctrl Pts',(-22.817839892186,193.502028447915,45.2081708191727));
#2181=CARTESIAN_POINT('Ctrl Pts',(-29.2444941385794,193.002028447915,40.5762979824596));
#2182=CARTESIAN_POINT('Ctrl Pts',(-35.6711483849729,192.502028447915,35.9444251457465));
#2183=CARTESIAN_POINT('Ctrl Pts',(-40.3519323616533,192.002028447915,29.5533069226325));
#2184=CARTESIAN_POINT('Ctrl Pts',(-45.0327163383337,191.502028447915,23.1621886995185));
#2185=CARTESIAN_POINT('Ctrl Pts',(-47.5094422967239,191.002028447915,15.6374322712211));
#2186=CARTESIAN_POINT('Ctrl Pts',(-49.9861682551141,190.502028447915,8.11267584292358));
#2187=CARTESIAN_POINT('Ctrl Pts',(-50.0163970020424,190.002028447915,0.190856796705288));
#2188=CARTESIAN_POINT('Ctrl Pts',(-50.0466257489707,189.502028447915,-7.73096224951301));
#2189=CARTESIAN_POINT('Ctrl Pts',(-47.6273982840717,189.002028447915,-15.2744010708495));
#2190=CARTESIAN_POINT('Ctrl Pts',(-45.2081708191727,188.502028447915,-22.817839892186));
#2191=CARTESIAN_POINT('Ctrl Pts',(-40.5762979824596,188.002028447915,-29.2444941385794));
#2192=CARTESIAN_POINT('Ctrl Pts',(-35.9444251457465,187.502028447915,-35.6711483849729));
#2193=CARTESIAN_POINT('Ctrl Pts',(-29.5533069226325,187.002028447915,-40.3519323616533));
#2194=CARTESIAN_POINT('Ctrl Pts',(-23.1621886995185,186.502028447915,-45.0327163383337));
#2195=CARTESIAN_POINT('Ctrl Pts',(-15.6374322712211,186.002028447915,-47.5094422967239));
#2196=CARTESIAN_POINT('Ctrl Pts',(-8.11267584292359,185.502028447915,-49.9861682551141));
#2197=CARTESIAN_POINT('Ctrl Pts',(-0.190856796705292,185.002028447915,-50.0163970020424));
#2198=CARTESIAN_POINT('Ctrl Pts',(7.730962249513,184.502028447915,-50.0466257489707));
#2199=CARTESIAN_POINT('Ctrl Pts',(15.2744010708495,184.002028447915,-47.6273982840717));
#2200=CARTESIAN_POINT('Ctrl Pts',(22.817839892186,183.502028447915,-45.2081708191727));
#2201=CARTESIAN_POINT('Ctrl Pts',(29.2444941385794,183.002028447915,-40.5762979824596));
#2202=CARTESIAN_POINT('Ctrl Pts',(35.6711483849729,182.502028447915,-35.9444251457465));
#2203=CARTESIAN_POINT('Ctrl Pts',(40.3519323616533,182.002028447915,-29.5533069226325));
#2204=CARTESIAN_POINT('Ctrl Pts',(45.0327163383337,181.502028447915,-23.1621886995185));
#2205=CARTESIAN_POINT('Ctrl Pts',(47.5094422967239,181.002028447915,-15.6374322712211));
#2206=CARTESIAN_POINT('Ctrl Pts',(49.9861682551141,180.502028447915,-8.11267584292359));
#2207=CARTESIAN_POINT('Ctrl Pts',(50.0163970020424,180.002028447915,-0.190856796705295));
#2208=CARTESIAN_POINT('Ctrl Pts',(50.0466257489707,179.502028447915,7.730962249513));
#2209=CARTESIAN_POINT('Ctrl Pts',(47.6273982840717,179.002028447915,15.2744010708495));
#2210=CARTESIAN_POINT('Ctrl Pts',(45.2081708191727,178.502028447915,22.817839892186));
#2211=CARTESIAN_POINT('Ctrl Pts',(40.5762979824596,178.002028447915,29.2444941385794));
#2212=CARTESIAN_POINT('Ctrl Pts',(35.9444251457465,177.502028447915,35.6711483849729));
#2213=CARTESIAN_POINT('Ctrl Pts',(29.5533069226325,177.002028447915,40.3519323616533));
#2214=CARTESIAN_POINT('Ctrl Pts',(23.1621886995185,176.502028447915,45.0327163383337));
#2215=CARTESIAN_POINT('Ctrl Pts',(15.6374322712211,176.002028447915,47.5094422967239));
#2216=CARTESIAN_POINT('Ctrl Pts',(8.11267584292359,175.502028447915,49.9861682551141));
#2217=CARTESIAN_POINT('Ctrl Pts',(0.190856796705285,175.002028447915,50.0163970020424));
#2218=CARTESIAN_POINT('Ctrl Pts',(0.000256710972400879,237.995967593475,
50.0163970020424));
#2219=CARTESIAN_POINT('Ctrl Pts',(-7.92156233524589,237.495967593475,50.0164376610661));
#2220=CARTESIAN_POINT('Ctrl Pts',(-15.4556725243922,236.995967593475,47.5684996184509));
#2221=CARTESIAN_POINT('Ctrl Pts',(-22.9897827135384,236.495967593475,45.1205615758357));
#2222=CARTESIAN_POINT('Ctrl Pts',(-29.3986928470667,235.995967593475,40.4642660629801));
#2223=CARTESIAN_POINT('Ctrl Pts',(-35.8076029805949,235.495967593475,35.8079705501245));
#2224=CARTESIAN_POINT('Ctrl Pts',(-40.4639642811328,234.995967593475,29.3991082141453));
#2225=CARTESIAN_POINT('Ctrl Pts',(-45.1203255816707,234.495967593475,22.990245878166));
#2226=CARTESIAN_POINT('Ctrl Pts',(-47.5683409623447,233.995967593475,15.4561608176784));
#2227=CARTESIAN_POINT('Ctrl Pts',(-50.0163563430187,233.495967593475,7.9220757571907));
#2228=CARTESIAN_POINT('Ctrl Pts',(-50.0163970020424,232.995967593475,0.000256710972403942));
#2229=CARTESIAN_POINT('Ctrl Pts',(-50.0164376610661,232.495967593475,-7.92156233524589));
#2230=CARTESIAN_POINT('Ctrl Pts',(-47.5684996184509,231.995967593475,-15.4556725243922));
#2231=CARTESIAN_POINT('Ctrl Pts',(-45.1205615758357,231.495967593475,-22.9897827135384));
#2232=CARTESIAN_POINT('Ctrl Pts',(-40.4642660629801,230.995967593475,-29.3986928470667));
#2233=CARTESIAN_POINT('Ctrl Pts',(-35.8079705501245,230.495967593475,-35.8076029805949));
#2234=CARTESIAN_POINT('Ctrl Pts',(-29.3991082141453,229.995967593475,-40.4639642811328));
#2235=CARTESIAN_POINT('Ctrl Pts',(-22.9902458781661,229.495967593475,-45.1203255816707));
#2236=CARTESIAN_POINT('Ctrl Pts',(-15.4561608176784,228.995967593475,-47.5683409623447));
#2237=CARTESIAN_POINT('Ctrl Pts',(-7.92207575719071,228.495967593475,-50.0163563430187));
#2238=CARTESIAN_POINT('Ctrl Pts',(-0.000256710972407005,227.995967593475,
-50.0163970020424));
#2239=CARTESIAN_POINT('Ctrl Pts',(7.92156233524589,227.495967593475,-50.0164376610661));
#2240=CARTESIAN_POINT('Ctrl Pts',(15.4556725243922,226.995967593475,-47.5684996184509));
#2241=CARTESIAN_POINT('Ctrl Pts',(22.9897827135384,226.495967593475,-45.1205615758357));
#2242=CARTESIAN_POINT('Ctrl Pts',(29.3986928470667,225.995967593475,-40.4642660629801));
#2243=CARTESIAN_POINT('Ctrl Pts',(35.8076029805949,225.495967593475,-35.8079705501245));
#2244=CARTESIAN_POINT('Ctrl Pts',(40.4639642811328,224.995967593475,-29.3991082141453));
#2245=CARTESIAN_POINT('Ctrl Pts',(45.1203255816707,224.495967593475,-22.9902458781661));
#2246=CARTESIAN_POINT('Ctrl Pts',(47.5683409623447,223.995967593475,-15.4561608176784));
#2247=CARTESIAN_POINT('Ctrl Pts',(50.0163563430187,223.495967593475,-7.92207575719071));
#2248=CARTESIAN_POINT('Ctrl Pts',(50.0163970020424,222.995967593475,-0.000256710972410067));
#2249=CARTESIAN_POINT('Ctrl Pts',(50.0164376610661,222.495967593475,7.92156233524589));
#2250=CARTESIAN_POINT('Ctrl Pts',(47.5684996184509,221.995967593475,15.4556725243922));
#2251=CARTESIAN_POINT('Ctrl Pts',(45.1205615758358,221.495967593475,22.9897827135384));
#2252=CARTESIAN_POINT('Ctrl Pts',(40.4642660629801,220.995967593475,29.3986928470667));
#2253=CARTESIAN_POINT('Ctrl Pts',(35.8079705501245,220.495967593475,35.8076029805949));
#2254=CARTESIAN_POINT('Ctrl Pts',(29.3991082141453,219.995967593475,40.4639642811328));
#2255=CARTESIAN_POINT('Ctrl Pts',(22.9902458781661,219.495967593475,45.1203255816707));
#2256=CARTESIAN_POINT('Ctrl Pts',(15.4561608176784,218.995967593475,47.5683409623447));
#2257=CARTESIAN_POINT('Ctrl Pts',(7.92207575719071,218.495967593475,50.0163563430187));
#2258=CARTESIAN_POINT('Ctrl Pts',(0.000256710972400879,217.995967593475,
50.0163970020424));
#2259=CARTESIAN_POINT('Ctrl Pts',(-7.92156233524589,217.495967593475,50.0164376610661));
#2260=CARTESIAN_POINT('Ctrl Pts',(-15.4556725243922,216.995967593475,47.5684996184509));
#2261=CARTESIAN_POINT('Ctrl Pts',(-22.9897827135384,216.495967593475,45.1205615758357));
#2262=CARTESIAN_POINT('Ctrl Pts',(-29.3986928470667,215.995967593475,40.4642660629801));
#2263=CARTESIAN_POINT('Ctrl Pts',(-35.8076029805949,215.495967593475,35.8079705501245));
#2264=CARTESIAN_POINT('Ctrl Pts',(-40.4639642811328,214.995967593475,29.3991082141453));
#2265=CARTESIAN_POINT('Ctrl Pts',(-45.1203255816707,214.495967593475,22.990245878166));
#2266=CARTESIAN_POINT('Ctrl Pts',(-47.5683409623447,213.995967593475,15.4561608176784));
#2267=CARTESIAN_POINT('Ctrl Pts',(-50.0163563430187,213.495967593475,7.9220757571907));
#2268=CARTESIAN_POINT('Ctrl Pts',(-50.0163970020424,212.995967593475,0.000256710972403942));
#2269=CARTESIAN_POINT('Ctrl Pts',(-50.0164376610661,212.495967593475,-7.92156233524589));
#2270=CARTESIAN_POINT('Ctrl Pts',(-47.5684996184509,211.995967593475,-15.4556725243922));
#2271=CARTESIAN_POINT('Ctrl Pts',(-45.1205615758357,211.495967593475,-22.9897827135384));
#2272=CARTESIAN_POINT('Ctrl Pts',(-40.4642660629801,210.995967593475,-29.3986928470667));
#2273=CARTESIAN_POINT('Ctrl Pts',(-35.8079705501245,210.495967593475,-35.8076029805949));
#2274=CARTESIAN_POINT('Ctrl Pts',(-29.3991082141453,209.995967593475,-40.4639642811328));
#2275=CARTESIAN_POINT('Ctrl Pts',(-22.9902458781661,209.495967593475,-45.1203255816707));
#2276=CARTESIAN_POINT('Ctrl Pts',(-15.4561608176784,208.995967593475,-47.5683409623447));
#2277=CARTESIAN_POINT('Ctrl Pts',(-7.92207575719071,208.495967593475,-50.0163563430187));
#2278=CARTESIAN_POINT('Ctrl Pts',(-0.000256710972407005,207.995967593475,
-50.0163970020424));
#2279=CARTESIAN_POINT('Ctrl Pts',(7.92156233524589,207.495967593475,-50.0164376610661));
#2280=CARTESIAN_POINT('Ctrl Pts',(15.4556725243922,206.995967593475,-47.5684996184509));
#2281=CARTESIAN_POINT('Ctrl Pts',(22.9897827135384,206.495967593475,-45.1205615758357));
#2282=CARTESIAN_POINT('Ctrl Pts',(29.3986928470667,205.995967593475,-40.4642660629801));
#2283=CARTESIAN_POINT('Ctrl Pts',(35.8076029805949,205.495967593475,-35.8079705501245));
#2284=CARTESIAN_POINT('Ctrl Pts',(40.4639642811328,204.995967593475,-29.3991082141453));
#2285=CARTESIAN_POINT('Ctrl Pts',(45.1203255816707,204.495967593475,-22.9902458781661));
#2286=CARTESIAN_POINT('Ctrl Pts',(47.5683409623447,203.995967593475,-15.4561608176784));
#2287=CARTESIAN_POINT('Ctrl Pts',(50.0163563430187,203.495967593475,-7.92207575719071));
#2288=CARTESIAN_POINT('Ctrl Pts',(50.0163970020424,202.995967593475,-0.000256710972410067));
#2289=CARTESIAN_POINT('Ctrl Pts',(50.0164376610661,202.495967593475,7.92156233524589));
#2290=CARTESIAN_POINT('Ctrl Pts',(47.5684996184509,201.995967593475,15.4556725243922));
#2291=CARTESIAN_POINT('Ctrl Pts',(45.1205615758358,201.495967593475,22.9897827135384));
#2292=CARTESIAN_POINT('Ctrl Pts',(40.4642660629801,200.995967593475,29.3986928470667));
#2293=CARTESIAN_POINT('Ctrl Pts',(35.8079705501245,200.495967593475,35.8076029805949));
#2294=CARTESIAN_POINT('Ctrl Pts',(29.3991082141453,199.995967593475,40.4639642811328));
#2295=CARTESIAN_POINT('Ctrl Pts',(22.9902458781661,199.495967593475,45.1203255816707));
#2296=CARTESIAN_POINT('Ctrl Pts',(15.4561608176784,198.995967593475,47.5683409623447));
#2297=CARTESIAN_POINT('Ctrl Pts',(7.92207575719071,198.495967593475,50.0163563430187));
#2298=CARTESIAN_POINT('Ctrl Pts',(0.000256710972400879,197.995967593475,
50.0163970020424));
#2299=CARTESIAN_POINT('Ctrl Pts',(-7.92156233524589,197.495967593475,50.0164376610661));
#2300=CARTESIAN_POINT('Ctrl Pts',(-15.4556725243922,196.995967593475,47.5684996184509));
#2301=CARTESIAN_POINT('Ctrl Pts',(-22.9897827135384,196.495967593475,45.1205615758357));
#2302=CARTESIAN_POINT('Ctrl Pts',(-29.3986928470667,195.995967593475,40.4642660629801));
#2303=CARTESIAN_POINT('Ctrl Pts',(-35.8076029805949,195.495967593475,35.8079705501245));
#2304=CARTESIAN_POINT('Ctrl Pts',(-40.4639642811328,194.995967593475,29.3991082141453));
#2305=CARTESIAN_POINT('Ctrl Pts',(-45.1203255816707,194.495967593475,22.990245878166));
#2306=CARTESIAN_POINT('Ctrl Pts',(-47.5683409623447,193.995967593475,15.4561608176784));
#2307=CARTESIAN_POINT('Ctrl Pts',(-50.0163563430187,193.495967593475,7.9220757571907));
#2308=CARTESIAN_POINT('Ctrl Pts',(-50.0163970020424,192.995967593475,0.000256710972403942));
#2309=CARTESIAN_POINT('Ctrl Pts',(-50.0164376610661,192.495967593475,-7.92156233524589));
#2310=CARTESIAN_POINT('Ctrl Pts',(-47.5684996184509,191.995967593475,-15.4556725243922));
#2311=CARTESIAN_POINT('Ctrl Pts',(-45.1205615758357,191.495967593475,-22.9897827135384));
#2312=CARTESIAN_POINT('Ctrl Pts',(-40.4642660629801,190.995967593475,-29.3986928470667));
#2313=CARTESIAN_POINT('Ctrl Pts',(-35.8079705501245,190.495967593475,-35.8076029805949));
#2314=CARTESIAN_POINT('Ctrl Pts',(-29.3991082141453,189.995967593475,-40.4639642811328));
#2315=CARTESIAN_POINT('Ctrl Pts',(-22.9902458781661,189.495967593475,-45.1203255816707));
#2316=CARTESIAN_POINT('Ctrl Pts',(-15.4561608176784,188.995967593475,-47.5683409623447));
#2317=CARTESIAN_POINT('Ctrl Pts',(-7.92207575719071,188.495967593475,-50.0163563430187));
#2318=CARTESIAN_POINT('Ctrl Pts',(-0.000256710972407005,187.995967593475,
-50.0163970020424));
#2319=CARTESIAN_POINT('Ctrl Pts',(7.92156233524589,187.495967593475,-50.0164376610661));
#2320=CARTESIAN_POINT('Ctrl Pts',(15.4556725243922,186.995967593475,-47.5684996184509));
#2321=CARTESIAN_POINT('Ctrl Pts',(22.9897827135384,186.495967593475,-45.1205615758357));
#2322=CARTESIAN_POINT('Ctrl Pts',(29.3986928470667,185.995967593475,-40.4642660629801));
#2323=CARTESIAN_POINT('Ctrl Pts',(35.8076029805949,185.495967593475,-35.8079705501245));
#2324=CARTESIAN_POINT('Ctrl Pts',(40.4639642811328,184.995967593475,-29.3991082141453));
#2325=CARTESIAN_POINT('Ctrl Pts',(45.1203255816707,184.495967593475,-22.9902458781661));
#2326=CARTESIAN_POINT('Ctrl Pts',(47.5683409623447,183.995967593475,-15.4561608176784));
#2327=CARTESIAN_POINT('Ctrl Pts',(50.0163563430187,183.495967593475,-7.92207575719071));
#2328=CARTESIAN_POINT('Ctrl Pts',(50.0163970020424,182.995967593475,-0.000256710972410067));
#2329=CARTESIAN_POINT('Ctrl Pts',(50.0164376610661,182.495967593475,7.92156233524589));
#2330=CARTESIAN_POINT('Ctrl Pts',(47.5684996184509,181.995967593475,15.4556725243922));
#2331=CARTESIAN_POINT('Ctrl Pts',(45.1205615758358,181.495967593475,22.9897827135384));
#2332=CARTESIAN_POINT('Ctrl Pts',(40.4642660629801,180.995967593475,29.3986928470667));
#2333=CARTESIAN_POINT('Ctrl Pts',(35.8079705501245,180.495967593475,35.8076029805949));
#2334=CARTESIAN_POINT('Ctrl Pts',(29.3991082141453,179.995967593475,40.4639642811328));
#2335=CARTESIAN_POINT('Ctrl Pts',(22.9902458781661,179.495967593475,45.1203255816707));
#2336=CARTESIAN_POINT('Ctrl Pts',(15.4561608176784,178.995967593475,47.5683409623447));
#2337=CARTESIAN_POINT('Ctrl Pts',(7.92207575719071,178.495967593475,50.0163563430187));
#2338=CARTESIAN_POINT('Ctrl Pts',(0.000256710972400879,177.995967593475,
50.0163970020424));
#2339=CARTESIAN_POINT('Ctrl Pts',(0.00025671097240121,237.995967593475,
7.5));
#2340=CARTESIAN_POINT('Ctrl Pts',(-1.18762659146162,237.495967593475,7.50004065902369));
#2341=CARTESIAN_POINT('Ctrl Pts',(-2.317383311169,236.995967593475,7.13300320026677));
#2342=CARTESIAN_POINT('Ctrl Pts',(-3.44714003087638,236.495967593475,6.76596574150984));
#2343=CARTESIAN_POINT('Ctrl Pts',(-4.40818170865423,235.995967593475,6.06777834873578));
#2344=CARTESIAN_POINT('Ctrl Pts',(-5.36922338643209,235.495967593475,5.36959095596173));
#2345=CARTESIAN_POINT('Ctrl Pts',(-6.06747656688843,234.995967593475,4.40859707573286));
#2346=CARTESIAN_POINT('Ctrl Pts',(-6.76572974734476,234.495967593475,3.447603195504));
#2347=CARTESIAN_POINT('Ctrl Pts',(-7.13284454416054,233.995967593475,2.31787160445521));
#2348=CARTESIAN_POINT('Ctrl Pts',(-7.49995934097631,233.495967593475,1.18814001340642));
#2349=CARTESIAN_POINT('Ctrl Pts',(-7.5,232.995967593475,0.000256710972401669));
#2350=CARTESIAN_POINT('Ctrl Pts',(-7.50004065902369,232.495967593475,-1.18762659146162));
#2351=CARTESIAN_POINT('Ctrl Pts',(-7.13300320026677,231.995967593475,-2.317383311169));
#2352=CARTESIAN_POINT('Ctrl Pts',(-6.76596574150984,231.495967593475,-3.44714003087638));
#2353=CARTESIAN_POINT('Ctrl Pts',(-6.06777834873578,230.995967593475,-4.40818170865423));
#2354=CARTESIAN_POINT('Ctrl Pts',(-5.36959095596173,230.495967593475,-5.36922338643209));
#2355=CARTESIAN_POINT('Ctrl Pts',(-4.40859707573286,229.995967593475,-6.06747656688843));
#2356=CARTESIAN_POINT('Ctrl Pts',(-3.447603195504,229.495967593475,-6.76572974734476));
#2357=CARTESIAN_POINT('Ctrl Pts',(-2.31787160445521,228.995967593475,-7.13284454416054));
#2358=CARTESIAN_POINT('Ctrl Pts',(-1.18814001340642,228.495967593475,-7.49995934097631));
#2359=CARTESIAN_POINT('Ctrl Pts',(-0.000256710972402128,227.995967593475,
-7.5));
#2360=CARTESIAN_POINT('Ctrl Pts',(1.18762659146162,227.495967593475,-7.50004065902369));
#2361=CARTESIAN_POINT('Ctrl Pts',(2.317383311169,226.995967593475,-7.13300320026677));
#2362=CARTESIAN_POINT('Ctrl Pts',(3.44714003087638,226.495967593475,-6.76596574150984));
#2363=CARTESIAN_POINT('Ctrl Pts',(4.40818170865423,225.995967593475,-6.06777834873578));
#2364=CARTESIAN_POINT('Ctrl Pts',(5.36922338643209,225.495967593475,-5.36959095596173));
#2365=CARTESIAN_POINT('Ctrl Pts',(6.06747656688843,224.995967593475,-4.40859707573286));
#2366=CARTESIAN_POINT('Ctrl Pts',(6.76572974734476,224.495967593475,-3.447603195504));
#2367=CARTESIAN_POINT('Ctrl Pts',(7.13284454416054,223.995967593475,-2.31787160445521));
#2368=CARTESIAN_POINT('Ctrl Pts',(7.49995934097631,223.495967593475,-1.18814001340642));
#2369=CARTESIAN_POINT('Ctrl Pts',(7.5,222.995967593475,-0.000256710972402588));
#2370=CARTESIAN_POINT('Ctrl Pts',(7.50004065902369,222.495967593475,1.18762659146162));
#2371=CARTESIAN_POINT('Ctrl Pts',(7.13300320026677,221.995967593475,2.317383311169));
#2372=CARTESIAN_POINT('Ctrl Pts',(6.76596574150984,221.495967593475,3.44714003087638));
#2373=CARTESIAN_POINT('Ctrl Pts',(6.06777834873579,220.995967593475,4.40818170865423));
#2374=CARTESIAN_POINT('Ctrl Pts',(5.36959095596173,220.495967593475,5.36922338643209));
#2375=CARTESIAN_POINT('Ctrl Pts',(4.40859707573286,219.995967593475,6.06747656688843));
#2376=CARTESIAN_POINT('Ctrl Pts',(3.447603195504,219.495967593475,6.76572974734476));
#2377=CARTESIAN_POINT('Ctrl Pts',(2.31787160445521,218.995967593475,7.13284454416054));
#2378=CARTESIAN_POINT('Ctrl Pts',(1.18814001340643,218.495967593475,7.49995934097631));
#2379=CARTESIAN_POINT('Ctrl Pts',(0.00025671097240121,217.995967593475,
7.5));
#2380=CARTESIAN_POINT('Ctrl Pts',(-1.18762659146162,217.495967593475,7.50004065902369));
#2381=CARTESIAN_POINT('Ctrl Pts',(-2.317383311169,216.995967593475,7.13300320026677));
#2382=CARTESIAN_POINT('Ctrl Pts',(-3.44714003087638,216.495967593475,6.76596574150984));
#2383=CARTESIAN_POINT('Ctrl Pts',(-4.40818170865423,215.995967593475,6.06777834873578));
#2384=CARTESIAN_POINT('Ctrl Pts',(-5.36922338643209,215.495967593475,5.36959095596173));
#2385=CARTESIAN_POINT('Ctrl Pts',(-6.06747656688843,214.995967593475,4.40859707573286));
#2386=CARTESIAN_POINT('Ctrl Pts',(-6.76572974734476,214.495967593475,3.447603195504));
#2387=CARTESIAN_POINT('Ctrl Pts',(-7.13284454416054,213.995967593475,2.31787160445521));
#2388=CARTESIAN_POINT('Ctrl Pts',(-7.49995934097631,213.495967593475,1.18814001340642));
#2389=CARTESIAN_POINT('Ctrl Pts',(-7.5,212.995967593475,0.000256710972401669));
#2390=CARTESIAN_POINT('Ctrl Pts',(-7.50004065902369,212.495967593475,-1.18762659146162));
#2391=CARTESIAN_POINT('Ctrl Pts',(-7.13300320026677,211.995967593475,-2.317383311169));
#2392=CARTESIAN_POINT('Ctrl Pts',(-6.76596574150984,211.495967593475,-3.44714003087638));
#2393=CARTESIAN_POINT('Ctrl Pts',(-6.06777834873578,210.995967593475,-4.40818170865423));
#2394=CARTESIAN_POINT('Ctrl Pts',(-5.36959095596173,210.495967593475,-5.36922338643209));
#2395=CARTESIAN_POINT('Ctrl Pts',(-4.40859707573286,209.995967593475,-6.06747656688843));
#2396=CARTESIAN_POINT('Ctrl Pts',(-3.447603195504,209.495967593475,-6.76572974734476));
#2397=CARTESIAN_POINT('Ctrl Pts',(-2.31787160445521,208.995967593475,-7.13284454416054));
#2398=CARTESIAN_POINT('Ctrl Pts',(-1.18814001340642,208.495967593475,-7.49995934097631));
#2399=CARTESIAN_POINT('Ctrl Pts',(-0.000256710972402128,207.995967593475,
-7.5));
#2400=CARTESIAN_POINT('Ctrl Pts',(1.18762659146162,207.495967593475,-7.50004065902369));
#2401=CARTESIAN_POINT('Ctrl Pts',(2.317383311169,206.995967593475,-7.13300320026677));
#2402=CARTESIAN_POINT('Ctrl Pts',(3.44714003087638,206.495967593475,-6.76596574150984));
#2403=CARTESIAN_POINT('Ctrl Pts',(4.40818170865423,205.995967593475,-6.06777834873578));
#2404=CARTESIAN_POINT('Ctrl Pts',(5.36922338643209,205.495967593475,-5.36959095596173));
#2405=CARTESIAN_POINT('Ctrl Pts',(6.06747656688843,204.995967593475,-4.40859707573286));
#2406=CARTESIAN_POINT('Ctrl Pts',(6.76572974734476,204.495967593475,-3.447603195504));
#2407=CARTESIAN_POINT('Ctrl Pts',(7.13284454416054,203.995967593475,-2.31787160445521));
#2408=CARTESIAN_POINT('Ctrl Pts',(7.49995934097631,203.495967593475,-1.18814001340642));
#2409=CARTESIAN_POINT('Ctrl Pts',(7.5,202.995967593475,-0.000256710972402588));
#2410=CARTESIAN_POINT('Ctrl Pts',(7.50004065902369,202.495967593475,1.18762659146162));
#2411=CARTESIAN_POINT('Ctrl Pts',(7.13300320026677,201.995967593475,2.317383311169));
#2412=CARTESIAN_POINT('Ctrl Pts',(6.76596574150984,201.495967593475,3.44714003087638));
#2413=CARTESIAN_POINT('Ctrl Pts',(6.06777834873579,200.995967593475,4.40818170865423));
#2414=CARTESIAN_POINT('Ctrl Pts',(5.36959095596173,200.495967593475,5.36922338643209));
#2415=CARTESIAN_POINT('Ctrl Pts',(4.40859707573286,199.995967593475,6.06747656688843));
#2416=CARTESIAN_POINT('Ctrl Pts',(3.447603195504,199.495967593475,6.76572974734476));
#2417=CARTESIAN_POINT('Ctrl Pts',(2.31787160445521,198.995967593475,7.13284454416054));
#2418=CARTESIAN_POINT('Ctrl Pts',(1.18814001340643,198.495967593475,7.49995934097631));
#2419=CARTESIAN_POINT('Ctrl Pts',(0.00025671097240121,197.995967593475,
7.5));
#2420=CARTESIAN_POINT('Ctrl Pts',(-1.18762659146162,197.495967593475,7.50004065902369));
#2421=CARTESIAN_POINT('Ctrl Pts',(-2.317383311169,196.995967593475,7.13300320026677));
#2422=CARTESIAN_POINT('Ctrl Pts',(-3.44714003087638,196.495967593475,6.76596574150984));
#2423=CARTESIAN_POINT('Ctrl Pts',(-4.40818170865423,195.995967593475,6.06777834873578));
#2424=CARTESIAN_POINT('Ctrl Pts',(-5.36922338643209,195.495967593475,5.36959095596173));
#2425=CARTESIAN_POINT('Ctrl Pts',(-6.06747656688843,194.995967593475,4.40859707573286));
#2426=CARTESIAN_POINT('Ctrl Pts',(-6.76572974734476,194.495967593475,3.447603195504));
#2427=CARTESIAN_POINT('Ctrl Pts',(-7.13284454416054,193.995967593475,2.31787160445521));
#2428=CARTESIAN_POINT('Ctrl Pts',(-7.49995934097631,193.495967593475,1.18814001340642));
#2429=CARTESIAN_POINT('Ctrl Pts',(-7.5,192.995967593475,0.000256710972401669));
#2430=CARTESIAN_POINT('Ctrl Pts',(-7.50004065902369,192.495967593475,-1.18762659146162));
#2431=CARTESIAN_POINT('Ctrl Pts',(-7.13300320026677,191.995967593475,-2.317383311169));
#2432=CARTESIAN_POINT('Ctrl Pts',(-6.76596574150984,191.495967593475,-3.44714003087638));
#2433=CARTESIAN_POINT('Ctrl Pts',(-6.06777834873578,190.995967593475,-4.40818170865423));
#2434=CARTESIAN_POINT('Ctrl Pts',(-5.36959095596173,190.495967593475,-5.36922338643209));
#2435=CARTESIAN_POINT('Ctrl Pts',(-4.40859707573286,189.995967593475,-6.06747656688843));
#2436=CARTESIAN_POINT('Ctrl Pts',(-3.447603195504,189.495967593475,-6.76572974734476));
#2437=CARTESIAN_POINT('Ctrl Pts',(-2.31787160445521,188.995967593475,-7.13284454416054));
#2438=CARTESIAN_POINT('Ctrl Pts',(-1.18814001340642,188.495967593475,-7.49995934097631));
#2439=CARTESIAN_POINT('Ctrl Pts',(-0.000256710972402128,187.995967593475,
-7.5));
#2440=CARTESIAN_POINT('Ctrl Pts',(1.18762659146162,187.495967593475,-7.50004065902369));
#2441=CARTESIAN_POINT('Ctrl Pts',(2.317383311169,186.995967593475,-7.13300320026677));
#2442=CARTESIAN_POINT('Ctrl Pts',(3.44714003087638,186.495967593475,-6.76596574150984));
#2443=CARTESIAN_POINT('Ctrl Pts',(4.40818170865423,185.995967593475,-6.06777834873578));
#2444=CARTESIAN_POINT('Ctrl Pts',(5.36922338643209,185.495967593475,-5.36959095596173));
#2445=CARTESIAN_POINT('Ctrl Pts',(6.06747656688843,184.995967593475,-4.40859707573286));
#2446=CARTESIAN_POINT('Ctrl Pts',(6.76572974734476,184.495967593475,-3.447603195504));
#2447=CARTESIAN_POINT('Ctrl Pts',(7.13284454416054,183.995967593475,-2.31787160445521));
#2448=CARTESIAN_POINT('Ctrl Pts',(7.49995934097631,183.495967593475,-1.18814001340642));
#2449=CARTESIAN_POINT('Ctrl Pts',(7.5,182.995967593475,-0.000256710972402588));
#2450=CARTESIAN_POINT('Ctrl Pts',(7.50004065902369,182.495967593475,1.18762659146162));
#2451=CARTESIAN_POINT('Ctrl Pts',(7.13300320026677,181.995967593475,2.317383311169));
#2452=CARTESIAN_POINT('Ctrl Pts',(6.76596574150984,181.495967593475,3.44714003087638));
#2453=CARTESIAN_POINT('Ctrl Pts',(6.06777834873579,180.995967593475,4.40818170865423));
#2454=CARTESIAN_POINT('Ctrl Pts',(5.36959095596173,180.495967593475,5.36922338643209));
#2455=CARTESIAN_POINT('Ctrl Pts',(4.40859707573286,179.995967593475,6.06747656688843));
#2456=CARTESIAN_POINT('Ctrl Pts',(3.447603195504,179.495967593475,6.76572974734476));
#2457=CARTESIAN_POINT('Ctrl Pts',(2.31787160445521,178.995967593475,7.13284454416054));
#2458=CARTESIAN_POINT('Ctrl Pts',(1.18814001340643,178.495967593475,7.49995934097631));
#2459=CARTESIAN_POINT('Ctrl Pts',(0.00025671097240121,177.995967593475,
7.5));
#2460=CARTESIAN_POINT('Ctrl Pts',(0.000256710972400845,237.995967593475,
50.0163970020424));
#2461=CARTESIAN_POINT('Ctrl Pts',(-7.92156233524589,237.495967593475,50.0164376610661));
#2462=CARTESIAN_POINT('Ctrl Pts',(-15.4556725243922,236.995967593475,47.5684996184509));
#2463=CARTESIAN_POINT('Ctrl Pts',(-22.9897827135384,236.495967593475,45.1205615758357));
#2464=CARTESIAN_POINT('Ctrl Pts',(-29.3986928470667,235.995967593475,40.4642660629801));
#2465=CARTESIAN_POINT('Ctrl Pts',(-35.8076029805949,235.495967593475,35.8079705501245));
#2466=CARTESIAN_POINT('Ctrl Pts',(-40.4639642811328,234.995967593475,29.3991082141453));
#2467=CARTESIAN_POINT('Ctrl Pts',(-45.1203255816707,234.495967593475,22.990245878166));
#2468=CARTESIAN_POINT('Ctrl Pts',(-47.5683409623447,233.995967593475,15.4561608176784));
#2469=CARTESIAN_POINT('Ctrl Pts',(-50.0163563430187,233.495967593475,7.9220757571907));
#2470=CARTESIAN_POINT('Ctrl Pts',(-50.0163970020424,232.995967593475,0.000256710972403907));
#2471=CARTESIAN_POINT('Ctrl Pts',(-50.0164376610661,232.495967593475,-7.92156233524589));
#2472=CARTESIAN_POINT('Ctrl Pts',(-47.5684996184509,231.995967593475,-15.4556725243922));
#2473=CARTESIAN_POINT('Ctrl Pts',(-45.1205615758357,231.495967593475,-22.9897827135384));
#2474=CARTESIAN_POINT('Ctrl Pts',(-40.4642660629801,230.995967593475,-29.3986928470667));
#2475=CARTESIAN_POINT('Ctrl Pts',(-35.8079705501245,230.495967593475,-35.8076029805949));
#2476=CARTESIAN_POINT('Ctrl Pts',(-29.3991082141453,229.995967593475,-40.4639642811328));
#2477=CARTESIAN_POINT('Ctrl Pts',(-22.9902458781661,229.495967593475,-45.1203255816707));
#2478=CARTESIAN_POINT('Ctrl Pts',(-15.4561608176784,228.995967593475,-47.5683409623447));
#2479=CARTESIAN_POINT('Ctrl Pts',(-7.92207575719071,228.495967593475,-50.0163563430187));
#2480=CARTESIAN_POINT('Ctrl Pts',(-0.00025671097240697,227.995967593475,
-50.0163970020424));
#2481=CARTESIAN_POINT('Ctrl Pts',(7.92156233524589,227.495967593475,-50.0164376610661));
#2482=CARTESIAN_POINT('Ctrl Pts',(15.4556725243922,226.995967593475,-47.5684996184509));
#2483=CARTESIAN_POINT('Ctrl Pts',(22.9897827135384,226.495967593475,-45.1205615758357));
#2484=CARTESIAN_POINT('Ctrl Pts',(29.3986928470667,225.995967593475,-40.4642660629801));
#2485=CARTESIAN_POINT('Ctrl Pts',(35.8076029805949,225.495967593475,-35.8079705501245));
#2486=CARTESIAN_POINT('Ctrl Pts',(40.4639642811328,224.995967593475,-29.3991082141453));
#2487=CARTESIAN_POINT('Ctrl Pts',(45.1203255816707,224.495967593475,-22.9902458781661));
#2488=CARTESIAN_POINT('Ctrl Pts',(47.5683409623447,223.995967593475,-15.4561608176784));
#2489=CARTESIAN_POINT('Ctrl Pts',(50.0163563430187,223.495967593475,-7.92207575719071));
#2490=CARTESIAN_POINT('Ctrl Pts',(50.0163970020424,222.995967593475,-0.000256710972410033));
#2491=CARTESIAN_POINT('Ctrl Pts',(50.0164376610661,222.495967593475,7.92156233524589));
#2492=CARTESIAN_POINT('Ctrl Pts',(47.5684996184509,221.995967593475,15.4556725243922));
#2493=CARTESIAN_POINT('Ctrl Pts',(45.1205615758358,221.495967593475,22.9897827135384));
#2494=CARTESIAN_POINT('Ctrl Pts',(40.4642660629801,220.995967593475,29.3986928470667));
#2495=CARTESIAN_POINT('Ctrl Pts',(35.8079705501245,220.495967593475,35.8076029805949));
#2496=CARTESIAN_POINT('Ctrl Pts',(29.3991082141453,219.995967593475,40.4639642811328));
#2497=CARTESIAN_POINT('Ctrl Pts',(22.9902458781661,219.495967593475,45.1203255816707));
#2498=CARTESIAN_POINT('Ctrl Pts',(15.4561608176784,218.995967593475,47.5683409623447));
#2499=CARTESIAN_POINT('Ctrl Pts',(7.92207575719071,218.495967593475,50.0163563430187));
#2500=CARTESIAN_POINT('Ctrl Pts',(0.000256710972400845,217.995967593475,
50.0163970020424));
#2501=CARTESIAN_POINT('Ctrl Pts',(-7.92156233524589,217.495967593475,50.0164376610661));
#2502=CARTESIAN_POINT('Ctrl Pts',(-15.4556725243922,216.995967593475,47.5684996184509));
#2503=CARTESIAN_POINT('Ctrl Pts',(-22.9897827135384,216.495967593475,45.1205615758357));
#2504=CARTESIAN_POINT('Ctrl Pts',(-29.3986928470667,215.995967593475,40.4642660629801));
#2505=CARTESIAN_POINT('Ctrl Pts',(-35.8076029805949,215.495967593475,35.8079705501245));
#2506=CARTESIAN_POINT('Ctrl Pts',(-40.4639642811328,214.995967593475,29.3991082141453));
#2507=CARTESIAN_POINT('Ctrl Pts',(-45.1203255816707,214.495967593475,22.990245878166));
#2508=CARTESIAN_POINT('Ctrl Pts',(-47.5683409623447,213.995967593475,15.4561608176784));
#2509=CARTESIAN_POINT('Ctrl Pts',(-50.0163563430187,213.495967593475,7.9220757571907));
#2510=CARTESIAN_POINT('Ctrl Pts',(-50.0163970020424,212.995967593475,0.000256710972403907));
#2511=CARTESIAN_POINT('Ctrl Pts',(-50.0164376610661,212.495967593475,-7.92156233524589));
#2512=CARTESIAN_POINT('Ctrl Pts',(-47.5684996184509,211.995967593475,-15.4556725243922));
#2513=CARTESIAN_POINT('Ctrl Pts',(-45.1205615758357,211.495967593475,-22.9897827135384));
#2514=CARTESIAN_POINT('Ctrl Pts',(-40.4642660629801,210.995967593475,-29.3986928470667));
#2515=CARTESIAN_POINT('Ctrl Pts',(-35.8079705501245,210.495967593475,-35.8076029805949));
#2516=CARTESIAN_POINT('Ctrl Pts',(-29.3991082141453,209.995967593475,-40.4639642811328));
#2517=CARTESIAN_POINT('Ctrl Pts',(-22.9902458781661,209.495967593475,-45.1203255816707));
#2518=CARTESIAN_POINT('Ctrl Pts',(-15.4561608176784,208.995967593475,-47.5683409623447));
#2519=CARTESIAN_POINT('Ctrl Pts',(-7.92207575719071,208.495967593475,-50.0163563430187));
#2520=CARTESIAN_POINT('Ctrl Pts',(-0.00025671097240697,207.995967593475,
-50.0163970020424));
#2521=CARTESIAN_POINT('Ctrl Pts',(7.92156233524589,207.495967593475,-50.0164376610661));
#2522=CARTESIAN_POINT('Ctrl Pts',(15.4556725243922,206.995967593475,-47.5684996184509));
#2523=CARTESIAN_POINT('Ctrl Pts',(22.9897827135384,206.495967593475,-45.1205615758357));
#2524=CARTESIAN_POINT('Ctrl Pts',(29.3986928470667,205.995967593475,-40.4642660629801));
#2525=CARTESIAN_POINT('Ctrl Pts',(35.8076029805949,205.495967593475,-35.8079705501245));
#2526=CARTESIAN_POINT('Ctrl Pts',(40.4639642811328,204.995967593475,-29.3991082141453));
#2527=CARTESIAN_POINT('Ctrl Pts',(45.1203255816707,204.495967593475,-22.9902458781661));
#2528=CARTESIAN_POINT('Ctrl Pts',(47.5683409623447,203.995967593475,-15.4561608176784));
#2529=CARTESIAN_POINT('Ctrl Pts',(50.0163563430187,203.495967593475,-7.92207575719071));
#2530=CARTESIAN_POINT('Ctrl Pts',(50.0163970020424,202.995967593475,-0.000256710972410033));
#2531=CARTESIAN_POINT('Ctrl Pts',(50.0164376610661,202.495967593475,7.92156233524589));
#2532=CARTESIAN_POINT('Ctrl Pts',(47.5684996184509,201.995967593475,15.4556725243922));
#2533=CARTESIAN_POINT('Ctrl Pts',(45.1205615758358,201.495967593475,22.9897827135384));
#2534=CARTESIAN_POINT('Ctrl Pts',(40.4642660629801,200.995967593475,29.3986928470667));
#2535=CARTESIAN_POINT('Ctrl Pts',(35.8079705501245,200.495967593475,35.8076029805949));
#2536=CARTESIAN_POINT('Ctrl Pts',(29.3991082141453,199.995967593475,40.4639642811328));
#2537=CARTESIAN_POINT('Ctrl Pts',(22.9902458781661,199.495967593475,45.1203255816707));
#2538=CARTESIAN_POINT('Ctrl Pts',(15.4561608176784,198.995967593475,47.5683409623447));
#2539=CARTESIAN_POINT('Ctrl Pts',(7.92207575719071,198.495967593475,50.0163563430187));
#2540=CARTESIAN_POINT('Ctrl Pts',(0.000256710972400845,197.995967593475,
50.0163970020424));
#2541=CARTESIAN_POINT('Ctrl Pts',(-7.92156233524589,197.495967593475,50.0164376610661));
#2542=CARTESIAN_POINT('Ctrl Pts',(-15.4556725243922,196.995967593475,47.5684996184509));
#2543=CARTESIAN_POINT('Ctrl Pts',(-22.9897827135384,196.495967593475,45.1205615758357));
#2544=CARTESIAN_POINT('Ctrl Pts',(-29.3986928470667,195.995967593475,40.4642660629801));
#2545=CARTESIAN_POINT('Ctrl Pts',(-35.8076029805949,195.495967593475,35.8079705501245));
#2546=CARTESIAN_POINT('Ctrl Pts',(-40.4639642811328,194.995967593475,29.3991082141453));
#2547=CARTESIAN_POINT('Ctrl Pts',(-45.1203255816707,194.495967593475,22.990245878166));
#2548=CARTESIAN_POINT('Ctrl Pts',(-47.5683409623447,193.995967593475,15.4561608176784));
#2549=CARTESIAN_POINT('Ctrl Pts',(-50.0163563430187,193.495967593475,7.9220757571907));
#2550=CARTESIAN_POINT('Ctrl Pts',(-50.0163970020424,192.995967593475,0.000256710972403907));
#2551=CARTESIAN_POINT('Ctrl Pts',(-50.0164376610661,192.495967593475,-7.92156233524589));
#2552=CARTESIAN_POINT('Ctrl Pts',(-47.5684996184509,191.995967593475,-15.4556725243922));
#2553=CARTESIAN_POINT('Ctrl Pts',(-45.1205615758357,191.495967593475,-22.9897827135384));
#2554=CARTESIAN_POINT('Ctrl Pts',(-40.4642660629801,190.995967593475,-29.3986928470667));
#2555=CARTESIAN_POINT('Ctrl Pts',(-35.8079705501245,190.495967593475,-35.8076029805949));
#2556=CARTESIAN_POINT('Ctrl Pts',(-29.3991082141453,189.995967593475,-40.4639642811328));
#2557=CARTESIAN_POINT('Ctrl Pts',(-22.9902458781661,189.495967593475,-45.1203255816707));
#2558=CARTESIAN_POINT('Ctrl Pts',(-15.4561608176784,188.995967593475,-47.5683409623447));
#2559=CARTESIAN_POINT('Ctrl Pts',(-7.92207575719071,188.495967593475,-50.0163563430187));
#2560=CARTESIAN_POINT('Ctrl Pts',(-0.00025671097240697,187.995967593475,
-50.0163970020424));
#2561=CARTESIAN_POINT('Ctrl Pts',(7.92156233524589,187.495967593475,-50.0164376610661));
#2562=CARTESIAN_POINT('Ctrl Pts',(15.4556725243922,186.995967593475,-47.5684996184509));
#2563=CARTESIAN_POINT('Ctrl Pts',(22.9897827135384,186.495967593475,-45.1205615758357));
#2564=CARTESIAN_POINT('Ctrl Pts',(29.3986928470667,185.995967593475,-40.4642660629801));
#2565=CARTESIAN_POINT('Ctrl Pts',(35.8076029805949,185.495967593475,-35.8079705501245));
#2566=CARTESIAN_POINT('Ctrl Pts',(40.4639642811328,184.995967593475,-29.3991082141453));
#2567=CARTESIAN_POINT('Ctrl Pts',(45.1203255816707,184.495967593475,-22.9902458781661));
#2568=CARTESIAN_POINT('Ctrl Pts',(47.5683409623447,183.995967593475,-15.4561608176784));
#2569=CARTESIAN_POINT('Ctrl Pts',(50.0163563430187,183.495967593475,-7.92207575719071));
#2570=CARTESIAN_POINT('Ctrl Pts',(50.0163970020424,182.995967593475,-0.000256710972410033));
#2571=CARTESIAN_POINT('Ctrl Pts',(50.0164376610661,182.495967593475,7.92156233524589));
#2572=CARTESIAN_POINT('Ctrl Pts',(47.5684996184509,181.995967593475,15.4556725243922));
#2573=CARTESIAN_POINT('Ctrl Pts',(45.1205615758358,181.495967593475,22.9897827135384));
#2574=CARTESIAN_POINT('Ctrl Pts',(40.4642660629801,180.995967593475,29.3986928470667));
#2575=CARTESIAN_POINT('Ctrl Pts',(35.8079705501245,180.495967593475,35.8076029805949));
#2576=CARTESIAN_POINT('Ctrl Pts',(29.3991082141453,179.995967593475,40.4639642811328));
#2577=CARTESIAN_POINT('Ctrl Pts',(22.9902458781661,179.495967593475,45.1203255816707));
#2578=CARTESIAN_POINT('Ctrl Pts',(15.4561608176784,178.995967593475,47.5683409623447));
#2579=CARTESIAN_POINT('Ctrl Pts',(7.92207575719071,178.495967593475,50.0163563430187));
#2580=CARTESIAN_POINT('Ctrl Pts',(0.000256710972400845,177.995967593475,
50.0163970020424));
#2581=CARTESIAN_POINT('Ctrl Pts',(0.190856796705285,235.002028447915,50.0163970020424));
#2582=CARTESIAN_POINT('Ctrl Pts',(-7.73096224951301,234.502028447915,50.0466257489707));
#2583=CARTESIAN_POINT('Ctrl Pts',(-15.2744010708495,234.002028447915,47.6273982840717));
#2584=CARTESIAN_POINT('Ctrl Pts',(-22.817839892186,233.502028447915,45.2081708191727));
#2585=CARTESIAN_POINT('Ctrl Pts',(-29.2444941385794,233.002028447915,40.5762979824596));
#2586=CARTESIAN_POINT('Ctrl Pts',(-35.6711483849729,232.502028447915,35.9444251457465));
#2587=CARTESIAN_POINT('Ctrl Pts',(-40.3519323616533,232.002028447915,29.5533069226325));
#2588=CARTESIAN_POINT('Ctrl Pts',(-45.0327163383337,231.502028447915,23.1621886995185));
#2589=CARTESIAN_POINT('Ctrl Pts',(-47.5094422967239,231.002028447915,15.6374322712211));
#2590=CARTESIAN_POINT('Ctrl Pts',(-49.9861682551141,230.502028447915,8.11267584292358));
#2591=CARTESIAN_POINT('Ctrl Pts',(-50.0163970020424,230.002028447915,0.190856796705288));
#2592=CARTESIAN_POINT('Ctrl Pts',(-50.0466257489707,229.502028447915,-7.73096224951301));
#2593=CARTESIAN_POINT('Ctrl Pts',(-47.6273982840717,229.002028447915,-15.2744010708495));
#2594=CARTESIAN_POINT('Ctrl Pts',(-45.2081708191727,228.502028447915,-22.817839892186));
#2595=CARTESIAN_POINT('Ctrl Pts',(-40.5762979824596,228.002028447915,-29.2444941385794));
#2596=CARTESIAN_POINT('Ctrl Pts',(-35.9444251457465,227.502028447915,-35.6711483849729));
#2597=CARTESIAN_POINT('Ctrl Pts',(-29.5533069226325,227.002028447915,-40.3519323616533));
#2598=CARTESIAN_POINT('Ctrl Pts',(-23.1621886995185,226.502028447915,-45.0327163383337));
#2599=CARTESIAN_POINT('Ctrl Pts',(-15.6374322712211,226.002028447915,-47.5094422967239));
#2600=CARTESIAN_POINT('Ctrl Pts',(-8.11267584292359,225.502028447915,-49.9861682551141));
#2601=CARTESIAN_POINT('Ctrl Pts',(-0.190856796705292,225.002028447915,-50.0163970020424));
#2602=CARTESIAN_POINT('Ctrl Pts',(7.730962249513,224.502028447915,-50.0466257489707));
#2603=CARTESIAN_POINT('Ctrl Pts',(15.2744010708495,224.002028447915,-47.6273982840717));
#2604=CARTESIAN_POINT('Ctrl Pts',(22.817839892186,223.502028447915,-45.2081708191727));
#2605=CARTESIAN_POINT('Ctrl Pts',(29.2444941385794,223.002028447915,-40.5762979824596));
#2606=CARTESIAN_POINT('Ctrl Pts',(35.6711483849729,222.502028447915,-35.9444251457465));
#2607=CARTESIAN_POINT('Ctrl Pts',(40.3519323616533,222.002028447915,-29.5533069226325));
#2608=CARTESIAN_POINT('Ctrl Pts',(45.0327163383337,221.502028447915,-23.1621886995185));
#2609=CARTESIAN_POINT('Ctrl Pts',(47.5094422967239,221.002028447915,-15.6374322712211));
#2610=CARTESIAN_POINT('Ctrl Pts',(49.9861682551141,220.502028447915,-8.11267584292359));
#2611=CARTESIAN_POINT('Ctrl Pts',(50.0163970020424,220.002028447915,-0.190856796705295));
#2612=CARTESIAN_POINT('Ctrl Pts',(50.0466257489707,219.502028447915,7.730962249513));
#2613=CARTESIAN_POINT('Ctrl Pts',(47.6273982840717,219.002028447915,15.2744010708495));
#2614=CARTESIAN_POINT('Ctrl Pts',(45.2081708191727,218.502028447915,22.817839892186));
#2615=CARTESIAN_POINT('Ctrl Pts',(40.5762979824596,218.002028447915,29.2444941385794));
#2616=CARTESIAN_POINT('Ctrl Pts',(35.9444251457465,217.502028447915,35.6711483849729));
#2617=CARTESIAN_POINT('Ctrl Pts',(29.5533069226325,217.002028447915,40.3519323616533));
#2618=CARTESIAN_POINT('Ctrl Pts',(23.1621886995185,216.502028447915,45.0327163383337));
#2619=CARTESIAN_POINT('Ctrl Pts',(15.6374322712211,216.002028447915,47.5094422967239));
#2620=CARTESIAN_POINT('Ctrl Pts',(8.11267584292359,215.502028447915,49.9861682551141));
#2621=CARTESIAN_POINT('Ctrl Pts',(0.190856796705285,215.002028447915,50.0163970020424));
#2622=CARTESIAN_POINT('Ctrl Pts',(-7.73096224951301,214.502028447915,50.0466257489707));
#2623=CARTESIAN_POINT('Ctrl Pts',(-15.2744010708495,214.002028447915,47.6273982840717));
#2624=CARTESIAN_POINT('Ctrl Pts',(-22.817839892186,213.502028447915,45.2081708191727));
#2625=CARTESIAN_POINT('Ctrl Pts',(-29.2444941385794,213.002028447915,40.5762979824596));
#2626=CARTESIAN_POINT('Ctrl Pts',(-35.6711483849729,212.502028447915,35.9444251457465));
#2627=CARTESIAN_POINT('Ctrl Pts',(-40.3519323616533,212.002028447915,29.5533069226325));
#2628=CARTESIAN_POINT('Ctrl Pts',(-45.0327163383337,211.502028447915,23.1621886995185));
#2629=CARTESIAN_POINT('Ctrl Pts',(-47.5094422967239,211.002028447915,15.6374322712211));
#2630=CARTESIAN_POINT('Ctrl Pts',(-49.9861682551141,210.502028447915,8.11267584292358));
#2631=CARTESIAN_POINT('Ctrl Pts',(-50.0163970020424,210.002028447915,0.190856796705288));
#2632=CARTESIAN_POINT('Ctrl Pts',(-50.0466257489707,209.502028447915,-7.73096224951301));
#2633=CARTESIAN_POINT('Ctrl Pts',(-47.6273982840717,209.002028447915,-15.2744010708495));
#2634=CARTESIAN_POINT('Ctrl Pts',(-45.2081708191727,208.502028447915,-22.817839892186));
#2635=CARTESIAN_POINT('Ctrl Pts',(-40.5762979824596,208.002028447915,-29.2444941385794));
#2636=CARTESIAN_POINT('Ctrl Pts',(-35.9444251457465,207.502028447915,-35.6711483849729));
#2637=CARTESIAN_POINT('Ctrl Pts',(-29.5533069226325,207.002028447915,-40.3519323616533));
#2638=CARTESIAN_POINT('Ctrl Pts',(-23.1621886995185,206.502028447915,-45.0327163383337));
#2639=CARTESIAN_POINT('Ctrl Pts',(-15.6374322712211,206.002028447915,-47.5094422967239));
#2640=CARTESIAN_POINT('Ctrl Pts',(-8.11267584292359,205.502028447915,-49.9861682551141));
#2641=CARTESIAN_POINT('Ctrl Pts',(-0.190856796705292,205.002028447915,-50.0163970020424));
#2642=CARTESIAN_POINT('Ctrl Pts',(7.730962249513,204.502028447915,-50.0466257489707));
#2643=CARTESIAN_POINT('Ctrl Pts',(15.2744010708495,204.002028447915,-47.6273982840717));
#2644=CARTESIAN_POINT('Ctrl Pts',(22.817839892186,203.502028447915,-45.2081708191727));
#2645=CARTESIAN_POINT('Ctrl Pts',(29.2444941385794,203.002028447915,-40.5762979824596));
#2646=CARTESIAN_POINT('Ctrl Pts',(35.6711483849729,202.502028447915,-35.9444251457465));
#2647=CARTESIAN_POINT('Ctrl Pts',(40.3519323616533,202.002028447915,-29.5533069226325));
#2648=CARTESIAN_POINT('Ctrl Pts',(45.0327163383337,201.502028447915,-23.1621886995185));
#2649=CARTESIAN_POINT('Ctrl Pts',(47.5094422967239,201.002028447915,-15.6374322712211));
#2650=CARTESIAN_POINT('Ctrl Pts',(49.9861682551141,200.502028447915,-8.11267584292359));
#2651=CARTESIAN_POINT('Ctrl Pts',(50.0163970020424,200.002028447915,-0.190856796705295));
#2652=CARTESIAN_POINT('Ctrl Pts',(50.0466257489707,199.502028447915,7.730962249513));
#2653=CARTESIAN_POINT('Ctrl Pts',(47.6273982840717,199.002028447915,15.2744010708495));
#2654=CARTESIAN_POINT('Ctrl Pts',(45.2081708191727,198.502028447915,22.817839892186));
#2655=CARTESIAN_POINT('Ctrl Pts',(40.5762979824596,198.002028447915,29.2444941385794));
#2656=CARTESIAN_POINT('Ctrl Pts',(35.9444251457465,197.502028447915,35.6711483849729));
#2657=CARTESIAN_POINT('Ctrl Pts',(29.5533069226325,197.002028447915,40.3519323616533));
#2658=CARTESIAN_POINT('Ctrl Pts',(23.1621886995185,196.502028447915,45.0327163383337));
#2659=CARTESIAN_POINT('Ctrl Pts',(15.6374322712211,196.002028447915,47.5094422967239));
#2660=CARTESIAN_POINT('Ctrl Pts',(8.11267584292359,195.502028447915,49.9861682551141));
#2661=CARTESIAN_POINT('Ctrl Pts',(0.190856796705285,195.002028447915,50.0163970020424));
#2662=CARTESIAN_POINT('Ctrl Pts',(-7.73096224951301,194.502028447915,50.0466257489707));
#2663=CARTESIAN_POINT('Ctrl Pts',(-15.2744010708495,194.002028447915,47.6273982840717));
#2664=CARTESIAN_POINT('Ctrl Pts',(-22.817839892186,193.502028447915,45.2081708191727));
#2665=CARTESIAN_POINT('Ctrl Pts',(-29.2444941385794,193.002028447915,40.5762979824596));
#2666=CARTESIAN_POINT('Ctrl Pts',(-35.6711483849729,192.502028447915,35.9444251457465));
#2667=CARTESIAN_POINT('Ctrl Pts',(-40.3519323616533,192.002028447915,29.5533069226325));
#2668=CARTESIAN_POINT('Ctrl Pts',(-45.0327163383337,191.502028447915,23.1621886995185));
#2669=CARTESIAN_POINT('Ctrl Pts',(-47.5094422967239,191.002028447915,15.6374322712211));
#2670=CARTESIAN_POINT('Ctrl Pts',(-49.9861682551141,190.502028447915,8.11267584292358));
#2671=CARTESIAN_POINT('Ctrl Pts',(-50.0163970020424,190.002028447915,0.190856796705288));
#2672=CARTESIAN_POINT('Ctrl Pts',(-50.0466257489707,189.502028447915,-7.73096224951301));
#2673=CARTESIAN_POINT('Ctrl Pts',(-47.6273982840717,189.002028447915,-15.2744010708495));
#2674=CARTESIAN_POINT('Ctrl Pts',(-45.2081708191727,188.502028447915,-22.817839892186));
#2675=CARTESIAN_POINT('Ctrl Pts',(-40.5762979824596,188.002028447915,-29.2444941385794));
#2676=CARTESIAN_POINT('Ctrl Pts',(-35.9444251457465,187.502028447915,-35.6711483849729));
#2677=CARTESIAN_POINT('Ctrl Pts',(-29.5533069226325,187.002028447915,-40.3519323616533));
#2678=CARTESIAN_POINT('Ctrl Pts',(-23.1621886995185,186.502028447915,-45.0327163383337));
#2679=CARTESIAN_POINT('Ctrl Pts',(-15.6374322712211,186.002028447915,-47.5094422967239));
#2680=CARTESIAN_POINT('Ctrl Pts',(-8.11267584292359,185.502028447915,-49.9861682551141));
#2681=CARTESIAN_POINT('Ctrl Pts',(-0.190856796705292,185.002028447915,-50.0163970020424));
#2682=CARTESIAN_POINT('Ctrl Pts',(7.730962249513,184.502028447915,-50.0466257489707));
#2683=CARTESIAN_POINT('Ctrl Pts',(15.2744010708495,184.002028447915,-47.6273982840717));
#2684=CARTESIAN_POINT('Ctrl Pts',(22.817839892186,183.502028447915,-45.2081708191727));
#2685=CARTESIAN_POINT('Ctrl Pts',(29.2444941385794,183.002028447915,-40.5762979824596));
#2686=CARTESIAN_POINT('Ctrl Pts',(35.6711483849729,182.502028447915,-35.9444251457465));
#2687=CARTESIAN_POINT('Ctrl Pts',(40.3519323616533,182.002028447915,-29.5533069226325));
#2688=CARTESIAN_POINT('Ctrl Pts',(45.0327163383337,181.502028447915,-23.1621886995185));
#2689=CARTESIAN_POINT('Ctrl Pts',(47.5094422967239,181.002028447915,-15.6374322712211));
#2690=CARTESIAN_POINT('Ctrl Pts',(49.9861682551141,180.502028447915,-8.11267584292359));
#2691=CARTESIAN_POINT('Ctrl Pts',(50.0163970020424,180.002028447915,-0.190856796705295));
#2692=CARTESIAN_POINT('Ctrl Pts',(50.0466257489707,179.502028447915,7.730962249513));
#2693=CARTESIAN_POINT('Ctrl Pts',(47.6273982840717,179.002028447915,15.2744010708495));
#2694=CARTESIAN_POINT('Ctrl Pts',(45.2081708191727,178.502028447915,22.817839892186));
#2695=CARTESIAN_POINT('Ctrl Pts',(40.5762979824596,178.002028447915,29.2444941385794));
#2696=CARTESIAN_POINT('Ctrl Pts',(35.9444251457465,177.502028447915,35.6711483849729));
#2697=CARTESIAN_POINT('Ctrl Pts',(29.5533069226325,177.002028447915,40.3519323616533));
#2698=CARTESIAN_POINT('Ctrl Pts',(23.1621886995185,176.502028447915,45.0327163383337));
#2699=CARTESIAN_POINT('Ctrl Pts',(15.6374322712211,176.002028447915,47.5094422967239));
#2700=CARTESIAN_POINT('Ctrl Pts',(8.11267584292359,175.502028447915,49.9861682551141));
#2701=CARTESIAN_POINT('Ctrl Pts',(0.190856796705285,175.002028447915,50.0163970020424));
#2702=CARTESIAN_POINT('Ctrl Pts',(0.000256710972400845,237.995967593475,
50.0163970020424));
#2703=CARTESIAN_POINT('Ctrl Pts',(-7.92156233524589,237.495967593475,50.0164376610661));
#2704=CARTESIAN_POINT('Ctrl Pts',(-15.4556725243922,236.995967593475,47.5684996184509));
#2705=CARTESIAN_POINT('Ctrl Pts',(-22.9897827135384,236.495967593475,45.1205615758357));
#2706=CARTESIAN_POINT('Ctrl Pts',(-29.3986928470667,235.995967593475,40.4642660629801));
#2707=CARTESIAN_POINT('Ctrl Pts',(-35.8076029805949,235.495967593475,35.8079705501245));
#2708=CARTESIAN_POINT('Ctrl Pts',(-40.4639642811328,234.995967593475,29.3991082141453));
#2709=CARTESIAN_POINT('Ctrl Pts',(-45.1203255816707,234.495967593475,22.990245878166));
#2710=CARTESIAN_POINT('Ctrl Pts',(-47.5683409623447,233.995967593475,15.4561608176784));
#2711=CARTESIAN_POINT('Ctrl Pts',(-50.0163563430187,233.495967593475,7.9220757571907));
#2712=CARTESIAN_POINT('Ctrl Pts',(-50.0163970020424,232.995967593475,0.000256710972403907));
#2713=CARTESIAN_POINT('Ctrl Pts',(-50.0164376610661,232.495967593475,-7.92156233524589));
#2714=CARTESIAN_POINT('Ctrl Pts',(-47.5684996184509,231.995967593475,-15.4556725243922));
#2715=CARTESIAN_POINT('Ctrl Pts',(-45.1205615758357,231.495967593475,-22.9897827135384));
#2716=CARTESIAN_POINT('Ctrl Pts',(-40.4642660629801,230.995967593475,-29.3986928470667));
#2717=CARTESIAN_POINT('Ctrl Pts',(-35.8079705501245,230.495967593475,-35.8076029805949));
#2718=CARTESIAN_POINT('Ctrl Pts',(-29.3991082141453,229.995967593475,-40.4639642811328));
#2719=CARTESIAN_POINT('Ctrl Pts',(-22.9902458781661,229.495967593475,-45.1203255816707));
#2720=CARTESIAN_POINT('Ctrl Pts',(-15.4561608176784,228.995967593475,-47.5683409623447));
#2721=CARTESIAN_POINT('Ctrl Pts',(-7.92207575719071,228.495967593475,-50.0163563430187));
#2722=CARTESIAN_POINT('Ctrl Pts',(-0.00025671097240697,227.995967593475,
-50.0163970020424));
#2723=CARTESIAN_POINT('Ctrl Pts',(7.92156233524589,227.495967593475,-50.0164376610661));
#2724=CARTESIAN_POINT('Ctrl Pts',(15.4556725243922,226.995967593475,-47.5684996184509));
#2725=CARTESIAN_POINT('Ctrl Pts',(22.9897827135384,226.495967593475,-45.1205615758357));
#2726=CARTESIAN_POINT('Ctrl Pts',(29.3986928470667,225.995967593475,-40.4642660629801));
#2727=CARTESIAN_POINT('Ctrl Pts',(35.8076029805949,225.495967593475,-35.8079705501245));
#2728=CARTESIAN_POINT('Ctrl Pts',(40.4639642811328,224.995967593475,-29.3991082141453));
#2729=CARTESIAN_POINT('Ctrl Pts',(45.1203255816707,224.495967593475,-22.9902458781661));
#2730=CARTESIAN_POINT('Ctrl Pts',(47.5683409623447,223.995967593475,-15.4561608176784));
#2731=CARTESIAN_POINT('Ctrl Pts',(50.0163563430187,223.495967593475,-7.92207575719071));
#2732=CARTESIAN_POINT('Ctrl Pts',(50.0163970020424,222.995967593475,-0.000256710972410033));
#2733=CARTESIAN_POINT('Ctrl Pts',(50.0164376610661,222.495967593475,7.92156233524589));
#2734=CARTESIAN_POINT('Ctrl Pts',(47.5684996184509,221.995967593475,15.4556725243922));
#2735=CARTESIAN_POINT('Ctrl Pts',(45.1205615758358,221.495967593475,22.9897827135384));
#2736=CARTESIAN_POINT('Ctrl Pts',(40.4642660629801,220.995967593475,29.3986928470667));
#2737=CARTESIAN_POINT('Ctrl Pts',(35.8079705501245,220.495967593475,35.8076029805949));
#2738=CARTESIAN_POINT('Ctrl Pts',(29.3991082141453,219.995967593475,40.4639642811328));
#2739=CARTESIAN_POINT('Ctrl Pts',(22.9902458781661,219.495967593475,45.1203255816707));
#2740=CARTESIAN_POINT('Ctrl Pts',(15.4561608176784,218.995967593475,47.5683409623447));
#2741=CARTESIAN_POINT('Ctrl Pts',(7.92207575719071,218.495967593475,50.0163563430187));
#2742=CARTESIAN_POINT('Ctrl Pts',(0.000256710972400845,217.995967593475,
50.0163970020424));
#2743=CARTESIAN_POINT('Ctrl Pts',(-7.92156233524589,217.495967593475,50.0164376610661));
#2744=CARTESIAN_POINT('Ctrl Pts',(-15.4556725243922,216.995967593475,47.5684996184509));
#2745=CARTESIAN_POINT('Ctrl Pts',(-22.9897827135384,216.495967593475,45.1205615758357));
#2746=CARTESIAN_POINT('Ctrl Pts',(-29.3986928470667,215.995967593475,40.4642660629801));
#2747=CARTESIAN_POINT('Ctrl Pts',(-35.8076029805949,215.495967593475,35.8079705501245));
#2748=CARTESIAN_POINT('Ctrl Pts',(-40.4639642811328,214.995967593475,29.3991082141453));
#2749=CARTESIAN_POINT('Ctrl Pts',(-45.1203255816707,214.495967593475,22.990245878166));
#2750=CARTESIAN_POINT('Ctrl Pts',(-47.5683409623447,213.995967593475,15.4561608176784));
#2751=CARTESIAN_POINT('Ctrl Pts',(-50.0163563430187,213.495967593475,7.9220757571907));
#2752=CARTESIAN_POINT('Ctrl Pts',(-50.0163970020424,212.995967593475,0.000256710972403907));
#2753=CARTESIAN_POINT('Ctrl Pts',(-50.0164376610661,212.495967593475,-7.92156233524589));
#2754=CARTESIAN_POINT('Ctrl Pts',(-47.5684996184509,211.995967593475,-15.4556725243922));
#2755=CARTESIAN_POINT('Ctrl Pts',(-45.1205615758357,211.495967593475,-22.9897827135384));
#2756=CARTESIAN_POINT('Ctrl Pts',(-40.4642660629801,210.995967593475,-29.3986928470667));
#2757=CARTESIAN_POINT('Ctrl Pts',(-35.8079705501245,210.495967593475,-35.8076029805949));
#2758=CARTESIAN_POINT('Ctrl Pts',(-29.3991082141453,209.995967593475,-40.4639642811328));
#2759=CARTESIAN_POINT('Ctrl Pts',(-22.9902458781661,209.495967593475,-45.1203255816707));
#2760=CARTESIAN_POINT('Ctrl Pts',(-15.4561608176784,208.995967593475,-47.5683409623447));
#2761=CARTESIAN_POINT('Ctrl Pts',(-7.92207575719071,208.495967593475,-50.0163563430187));
#2762=CARTESIAN_POINT('Ctrl Pts',(-0.00025671097240697,207.995967593475,
-50.0163970020424));
#2763=CARTESIAN_POINT('Ctrl Pts',(7.92156233524589,207.495967593475,-50.0164376610661));
#2764=CARTESIAN_POINT('Ctrl Pts',(15.4556725243922,206.995967593475,-47.5684996184509));
#2765=CARTESIAN_POINT('Ctrl Pts',(22.9897827135384,206.495967593475,-45.1205615758357));
#2766=CARTESIAN_POINT('Ctrl Pts',(29.3986928470667,205.995967593475,-40.4642660629801));
#2767=CARTESIAN_POINT('Ctrl Pts',(35.8076029805949,205.495967593475,-35.8079705501245));
#2768=CARTESIAN_POINT('Ctrl Pts',(40.4639642811328,204.995967593475,-29.3991082141453));
#2769=CARTESIAN_POINT('Ctrl Pts',(45.1203255816707,204.495967593475,-22.9902458781661));
#2770=CARTESIAN_POINT('Ctrl Pts',(47.5683409623447,203.995967593475,-15.4561608176784));
#2771=CARTESIAN_POINT('Ctrl Pts',(50.0163563430187,203.495967593475,-7.92207575719071));
#2772=CARTESIAN_POINT('Ctrl Pts',(50.0163970020424,202.995967593475,-0.000256710972410033));
#2773=CARTESIAN_POINT('Ctrl Pts',(50.0164376610661,202.495967593475,7.92156233524589));
#2774=CARTESIAN_POINT('Ctrl Pts',(47.5684996184509,201.995967593475,15.4556725243922));
#2775=CARTESIAN_POINT('Ctrl Pts',(45.1205615758358,201.495967593475,22.9897827135384));
#2776=CARTESIAN_POINT('Ctrl Pts',(40.4642660629801,200.995967593475,29.3986928470667));
#2777=CARTESIAN_POINT('Ctrl Pts',(35.8079705501245,200.495967593475,35.8076029805949));
#2778=CARTESIAN_POINT('Ctrl Pts',(29.3991082141453,199.995967593475,40.4639642811328));
#2779=CARTESIAN_POINT('Ctrl Pts',(22.9902458781661,199.495967593475,45.1203255816707));
#2780=CARTESIAN_POINT('Ctrl Pts',(15.4561608176784,198.995967593475,47.5683409623447));
#2781=CARTESIAN_POINT('Ctrl Pts',(7.92207575719071,198.495967593475,50.0163563430187));
#2782=CARTESIAN_POINT('Ctrl Pts',(0.000256710972400845,197.995967593475,
50.0163970020424));
#2783=CARTESIAN_POINT('Ctrl Pts',(-7.92156233524589,197.495967593475,50.0164376610661));
#2784=CARTESIAN_POINT('Ctrl Pts',(-15.4556725243922,196.995967593475,47.5684996184509));
#2785=CARTESIAN_POINT('Ctrl Pts',(-22.9897827135384,196.495967593475,45.1205615758357));
#2786=CARTESIAN_POINT('Ctrl Pts',(-29.3986928470667,195.995967593475,40.4642660629801));
#2787=CARTESIAN_POINT('Ctrl Pts',(-35.8076029805949,195.495967593475,35.8079705501245));
#2788=CARTESIAN_POINT('Ctrl Pts',(-40.4639642811328,194.995967593475,29.3991082141453));
#2789=CARTESIAN_POINT('Ctrl Pts',(-45.1203255816707,194.495967593475,22.990245878166));
#2790=CARTESIAN_POINT('Ctrl Pts',(-47.5683409623447,193.995967593475,15.4561608176784));
#2791=CARTESIAN_POINT('Ctrl Pts',(-50.0163563430187,193.495967593475,7.9220757571907));
#2792=CARTESIAN_POINT('Ctrl Pts',(-50.0163970020424,192.995967593475,0.000256710972403907));
#2793=CARTESIAN_POINT('Ctrl Pts',(-50.0164376610661,192.495967593475,-7.92156233524589));
#2794=CARTESIAN_POINT('Ctrl Pts',(-47.5684996184509,191.995967593475,-15.4556725243922));
#2795=CARTESIAN_POINT('Ctrl Pts',(-45.1205615758357,191.495967593475,-22.9897827135384));
#2796=CARTESIAN_POINT('Ctrl Pts',(-40.4642660629801,190.995967593475,-29.3986928470667));
#2797=CARTESIAN_POINT('Ctrl Pts',(-35.8079705501245,190.495967593475,-35.8076029805949));
#2798=CARTESIAN_POINT('Ctrl Pts',(-29.3991082141453,189.995967593475,-40.4639642811328));
#2799=CARTESIAN_POINT('Ctrl Pts',(-22.9902458781661,189.495967593475,-45.1203255816707));
#2800=CARTESIAN_POINT('Ctrl Pts',(-15.4561608176784,188.995967593475,-47.5683409623447));
#2801=CARTESIAN_POINT('Ctrl Pts',(-7.92207575719071,188.495967593475,-50.0163563430187));
#2802=CARTESIAN_POINT('Ctrl Pts',(-0.00025671097240697,187.995967593475,
-50.0163970020424));
#2803=CARTESIAN_POINT('Ctrl Pts',(7.92156233524589,187.495967593475,-50.0164376610661));
#2804=CARTESIAN_POINT('Ctrl Pts',(15.4556725243922,186.995967593475,-47.5684996184509));
#2805=CARTESIAN_POINT('Ctrl Pts',(22.9897827135384,186.495967593475,-45.1205615758357));
#2806=CARTESIAN_POINT('Ctrl Pts',(29.3986928470667,185.995967593475,-40.4642660629801));
#2807=CARTESIAN_POINT('Ctrl Pts',(35.8076029805949,185.495967593475,-35.8079705501245));
#2808=CARTESIAN_POINT('Ctrl Pts',(40.4639642811328,184.995967593475,-29.3991082141453));
#2809=CARTESIAN_POINT('Ctrl Pts',(45.1203255816707,184.495967593475,-22.9902458781661));
#2810=CARTESIAN_POINT('Ctrl Pts',(47.5683409623447,183.995967593475,-15.4561608176784));
#2811=CARTESIAN_POINT('Ctrl Pts',(50.0163563430187,183.495967593475,-7.92207575719071));
#2812=CARTESIAN_POINT('Ctrl Pts',(50.0163970020424,182.995967593475,-0.000256710972410033));
#2813=CARTESIAN_POINT('Ctrl Pts',(50.0164376610661,182.495967593475,7.92156233524589));
#2814=CARTESIAN_POINT('Ctrl Pts',(47.5684996184509,181.995967593475,15.4556725243922));
#2815=CARTESIAN_POINT('Ctrl Pts',(45.1205615758358,181.495967593475,22.9897827135384));
#2816=CARTESIAN_POINT('Ctrl Pts',(40.4642660629801,180.995967593475,29.3986928470667));
#2817=CARTESIAN_POINT('Ctrl Pts',(35.8079705501245,180.495967593475,35.8076029805949));
#2818=CARTESIAN_POINT('Ctrl Pts',(29.3991082141453,179.995967593475,40.4639642811328));
#2819=CARTESIAN_POINT('Ctrl Pts',(22.9902458781661,179.495967593475,45.1203255816707));
#2820=CARTESIAN_POINT('Ctrl Pts',(15.4561608176784,178.995967593475,47.5683409623447));
#2821=CARTESIAN_POINT('Ctrl Pts',(7.92207575719071,178.495967593475,50.0163563430187));
#2822=CARTESIAN_POINT('Ctrl Pts',(0.000256710972400845,177.995967593475,
50.0163970020424));
#2823=CARTESIAN_POINT('Origin',(0.,150.,0.));
#2824=CARTESIAN_POINT('',(-5.,100.,-24.4948974278318));
#2825=CARTESIAN_POINT('',(5.,100.,-24.4948974278318));
#2826=CARTESIAN_POINT('Origin',(0.,100.,0.));
#2827=CARTESIAN_POINT('',(5.,150.,-24.4948974278318));
#2828=CARTESIAN_POINT('',(5.,150.,-24.4948974278318));
#2829=CARTESIAN_POINT('',(-5.,150.,-24.4948974278318));
#2830=CARTESIAN_POINT('Origin',(0.,150.,0.));
#2831=CARTESIAN_POINT('',(-5.,150.,-24.4948974278318));
#2832=CARTESIAN_POINT('Origin',(5.,150.,-33.));
#2833=CARTESIAN_POINT('',(5.,100.,-33.));
#2834=CARTESIAN_POINT('',(5.,100.,-24.4948974278318));
#2835=CARTESIAN_POINT('',(5.,150.,-33.));
#2836=CARTESIAN_POINT('',(5.,150.,-33.));
#2837=CARTESIAN_POINT('',(5.,150.,-24.4948974278318));
#2838=CARTESIAN_POINT('Origin',(-5.,150.,-33.));
#2839=CARTESIAN_POINT('',(-5.,100.,-33.));
#2840=CARTESIAN_POINT('',(5.,100.,-33.));
#2841=CARTESIAN_POINT('',(-5.,150.,-33.));
#2842=CARTESIAN_POINT('',(-5.,150.,-33.));
#2843=CARTESIAN_POINT('',(5.,150.,-33.));
#2844=CARTESIAN_POINT('Origin',(-5.,150.,-33.));
#2845=CARTESIAN_POINT('',(-5.,100.,-33.));
#2846=CARTESIAN_POINT('',(-5.,150.,-33.));
#2847=CARTESIAN_POINT('Origin',(0.,150.,0.));
#2848=CARTESIAN_POINT('Origin',(0.,100.,0.));
#2853=UNCERTAINTY_MEASURE_WITH_UNIT(LENGTH_MEASURE(0.01),#2859,
'DISTANCE_ACCURACY_VALUE',
'Maximum model space distance between geometric entities at asserted c
onnectivities');
#2854=UNCERTAINTY_MEASURE_WITH_UNIT(LENGTH_MEASURE(0.01),#2859,
'DISTANCE_ACCURACY_VALUE',
'Maximum model space distance between geometric entities at asserted c
onnectivities');
#2857=(
GEOMETRIC_REPRESENTATION_CONTEXT(3)
GLOBAL_UNCERTAINTY_ASSIGNED_CONTEXT((#2853))
GLOBAL_UNIT_ASSIGNED_CONTEXT((#2859,#2861,#2862))
REPRESENTATION_CONTEXT('','3D')
);
#2858=(
GEOMETRIC_REPRESENTATION_CONTEXT(3)
GLOBAL_UNCERTAINTY_ASSIGNED_CONTEXT((#2854))
GLOBAL_UNIT_ASSIGNED_CONTEXT((#2859,#2861,#2862))
REPRESENTATION_CONTEXT('','3D')
);
#2859=(
LENGTH_UNIT()
NAMED_UNIT(*)
SI_UNIT(.MILLI.,.METRE.)
);
#2861=(
NAMED_UNIT(*)
PLANE_ANGLE_UNIT()
SI_UNIT($,.RADIAN.)
);
#2862=(
NAMED_UNIT(*)
SI_UNIT($,.STERADIAN.)
SOLID_ANGLE_UNIT()
);
#2865=SHAPE_DEFINITION_REPRESENTATION(#2868,#2873);
#2868=PRODUCT_DEFINITION_SHAPE('',$,#2877);
#2873=SHAPE_REPRESENTATION('',(#434),#2857);
#2874=PRODUCT_DEFINITION_CONTEXT('part definition',#2885,'design');
#2877=PRODUCT_DEFINITION('Screw Feeder','Screw Feeder',#2880,#2874);
#2880=PRODUCT_DEFINITION_FORMATION('',$,#2889);
#2885=APPLICATION_CONTEXT(
'Core Data for Automotive Mechanical Design Process');
#2886=PRODUCT_CONTEXT('part definition',#2885,'mechanical');
#2889=PRODUCT('Screw Feeder','Screw Feeder',$,(#2886));
#2890=PRESENTATION_STYLE_ASSIGNMENT((#2891));
#2891=SURFACE_STYLE_USAGE(.BOTH.,#2892);
#2892=SURFACE_SIDE_STYLE('',(#2893));
#2893=SURFACE_STYLE_FILL_AREA(#2894);
#2894=FILL_AREA_STYLE('Steel - Satin',(#2895));
#2895=FILL_AREA_STYLE_COLOUR('Steel - Satin',#2896);
#2896=COLOUR_RGB('Steel - Satin',0.627450980392157,0.627450980392157,0.627450980392157);
ENDSEC;
END-ISO-10303-21;
